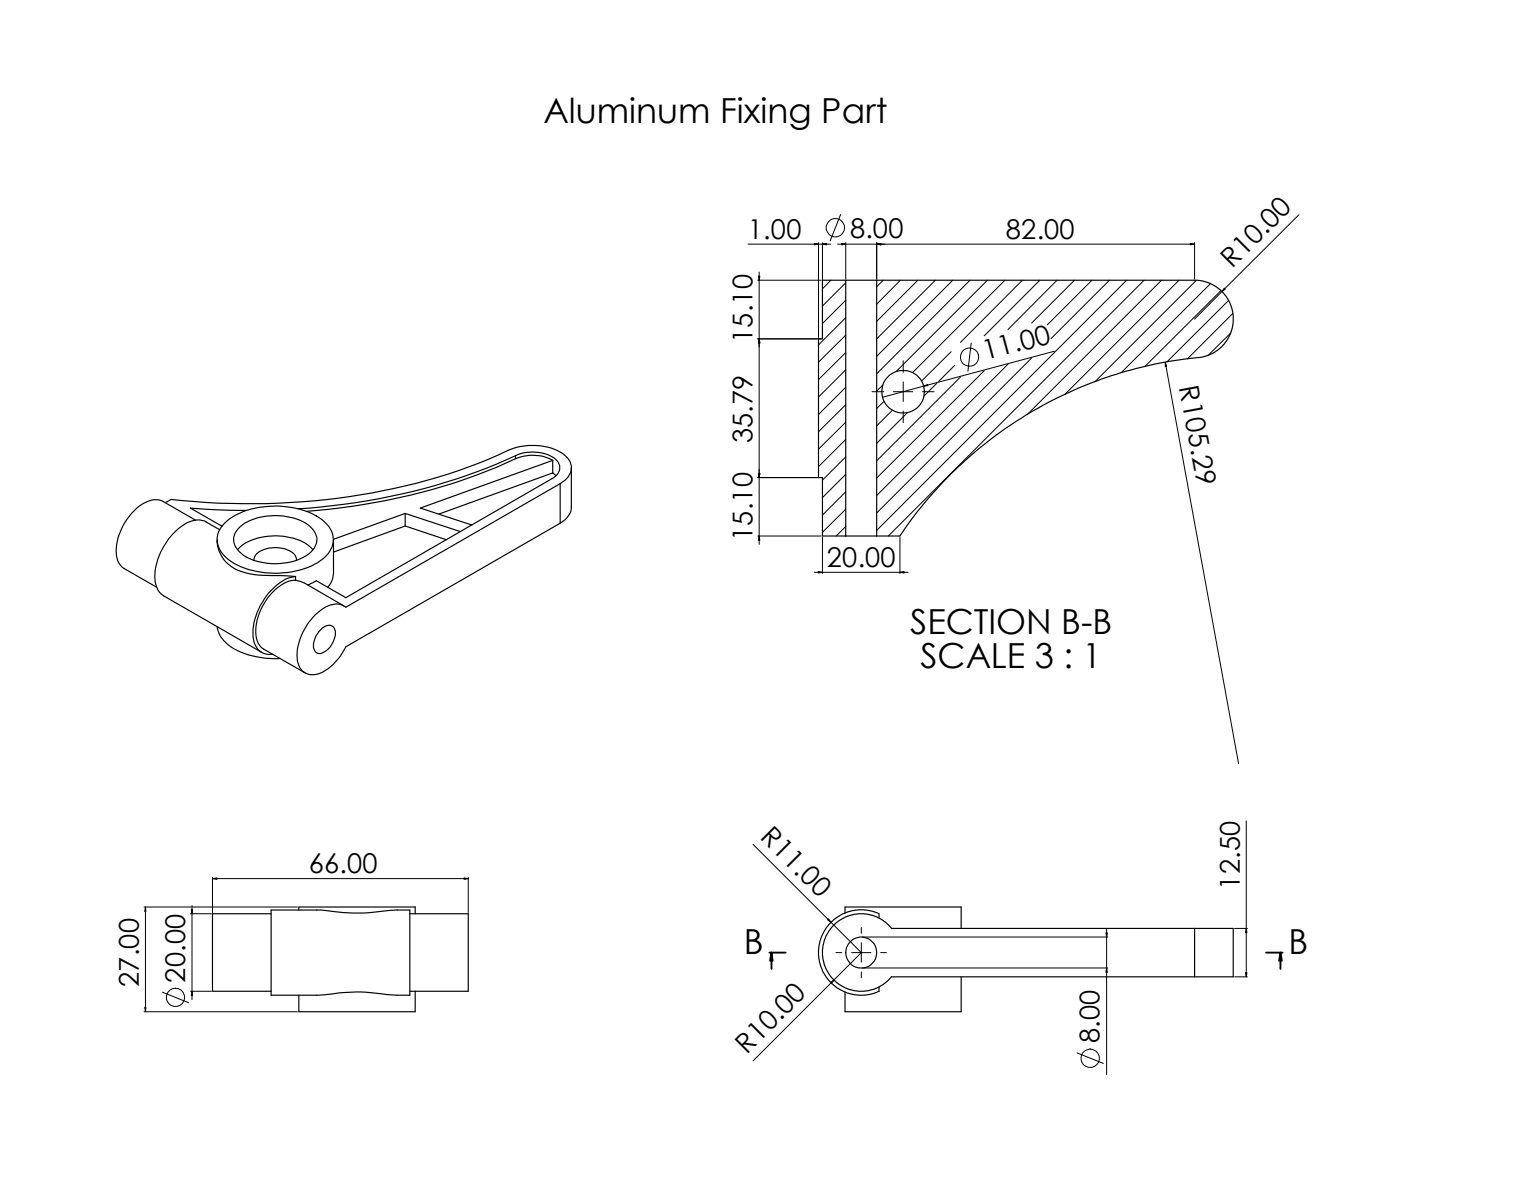
ISO-10303-21;
HEADER;
FILE_DESCRIPTION (('STEP AP214'),
    '1' );
FILE_NAME ('Aluminum Fixing Part.step',
    '2026-10-25T21:42:00',
    ( '' ),
    ( '' ),
    'SwSTEP 2.0',
    'SolidWorks 2025',
    '' );
FILE_SCHEMA (( 'AUTOMOTIVE_DESIGN' ));
ENDSEC;

DATA;
#1=ORIENTED_EDGE ( 'NONE', *, *, #7735, .T. ) ;
#6=CARTESIAN_POINT ( 'NONE',  ( 18.72350467417358288, 2.811787160796888063, 33.16867180916269575 ) ) ;
#84=DIRECTION ( 'NONE',  ( 0.9643627188534427130, 0.000000000000000000, -0.2645837230171117493 ) ) ;
#98=CARTESIAN_POINT ( 'NONE',  ( 4.257384923554910827, 7.250000000000000000, 44.19375250200204164 ) ) ;
#119=( LENGTH_UNIT ( ) NAMED_UNIT ( * ) SI_UNIT ( .MILLI., .METRE. ) );
#157=DIRECTION ( 'NONE',  ( 0.000000000000000000, -1.000000000000000000, 0.000000000000000000 ) ) ;
#171=DIRECTION ( 'NONE',  ( 0.000000000000000000, 0.000000000000000000, 1.000000000000000000 ) ) ;
#189=CARTESIAN_POINT ( 'NONE',  ( 4.257384923554910827, 5.669190722567434726, 44.19375250200204164 ) ) ;
#202=EDGE_LOOP ( 'NONE', ( #15560, #16098, #14916, #31484, #39561 ) ) ;
#206=ORIENTED_EDGE ( 'NONE', *, *, #8749, .F. ) ;
#214=CARTESIAN_POINT ( 'NONE',  ( -2.668805347656625298E-15, -4.500000000000000000, 40.00000000000002132 ) ) ;
#223=VERTEX_POINT ( 'NONE', #2823 ) ;
#248=CARTESIAN_POINT ( 'NONE',  ( 30.00000000000000000, 21.91020392607983780, -13.91584042252958930 ) ) ;
#255=ORIENTED_EDGE ( 'NONE', *, *, #34285, .F. ) ;
#303=ORIENTED_EDGE ( 'NONE', *, *, #35020, .T. ) ;
#331=( NAMED_UNIT ( * ) SI_UNIT ( $, .STERADIAN. ) SOLID_ANGLE_UNIT ( ) );
#338=EDGE_CURVE ( 'NONE', #35065, #41070, #33507, .T. ) ;
#384=LINE ( 'NONE', #32919, #10892 ) ;
#399=CARTESIAN_POINT ( 'NONE',  ( 8.846224670336669149, -14.93588149077679006, 43.47904789183715479 ) ) ;
#437=ORIENTED_EDGE ( 'NONE', *, *, #42084, .T. ) ;
#463=CARTESIAN_POINT ( 'NONE',  ( -26.68952268848979870, -10.75000000000000000, 29.19375250200205230 ) ) ;
#479=ORIENTED_EDGE ( 'NONE', *, *, #8404, .T. ) ;
#515=DIRECTION ( 'NONE',  ( -0.000000000000000000, 1.000000000000000000, -0.000000000000000000 ) ) ;
#522=PRODUCT_CONTEXT ( 'NONE', #9527, 'mechanical' ) ;
#528=EDGE_LOOP ( 'NONE', ( #25720, #24878, #1086, #1385 ) ) ;
#534=EDGE_CURVE ( 'NONE', #29227, #21343, #35976, .T. ) ;
#535=ORIENTED_EDGE ( 'NONE', *, *, #30609, .T. ) ;
#569=VERTEX_POINT ( 'NONE', #13431 ) ;
#579=DIRECTION ( 'NONE',  ( 0.000000000000000000, 1.000000000000000000, 0.000000000000000000 ) ) ;
#623=ORIENTED_EDGE ( 'NONE', *, *, #27491, .F. ) ;
#670=DIRECTION ( 'NONE',  ( 0.000000000000000000, -0.000000000000000000, 1.000000000000000000 ) ) ;
#675=LINE ( 'NONE', #32171, #20640 ) ;
#684=EDGE_CURVE ( 'NONE', #35318, #5713, #28096, .T. ) ;
#732=EDGE_CURVE ( 'NONE', #4073, #42083, #27874, .T. ) ;
#738=VECTOR ( 'NONE', #22456, 1000.000000000000000 ) ;
#761=CARTESIAN_POINT ( 'NONE',  ( 17.89728711128010730, -14.50803179344132410, 35.43499182679077109 ) ) ;
#780=CARTESIAN_POINT ( 'NONE',  ( 13.04894127963215666, -10.75000000000000000, -46.98814490019994139 ) ) ;
#788=ORIENTED_EDGE ( 'NONE', *, *, #20511, .T. ) ;
#802=VERTEX_POINT ( 'NONE', #2351 ) ;
#828=CARTESIAN_POINT ( 'NONE',  ( 15.87547634500077720, -15.42497640701065009, 38.68845844545155188 ) ) ;
#848=DIRECTION ( 'NONE',  ( 1.000000000000000000, 0.000000000000000000, 2.102695122396128930E-16 ) ) ;
#868=CIRCLE ( 'NONE', #30073, 14.99999999999999822 ) ;
#905=EDGE_CURVE ( 'NONE', #16080, #12680, #8463, .T. ) ;
#914=DIRECTION ( 'NONE',  ( 0.000000000000000000, 0.000000000000000000, -1.000000000000000000 ) ) ;
#956=DIRECTION ( 'NONE',  ( 0.000000000000000000, 0.000000000000000000, 1.000000000000000000 ) ) ;
#965=CARTESIAN_POINT ( 'NONE',  ( 18.48006385112488914, -12.48392328919574723, 33.96838569447678680 ) ) ;
#1041=CARTESIAN_POINT ( 'NONE',  ( 4.257384923554910827, 7.250000000000000000, 18.45625250200204448 ) ) ;
#1064=EDGE_LOOP ( 'NONE', ( #30938, #17529, #27633, #33315, #32704 ) ) ;
#1065=CARTESIAN_POINT ( 'NONE',  ( 33.00000000000001421, -4.500000000000000000, 44.00000000000003553 ) ) ;
#1086=ORIENTED_EDGE ( 'NONE', *, *, #29539, .F. ) ;
#1108=CARTESIAN_POINT ( 'NONE',  ( -91.72768752788732627, 1.750000000000001554, -57.39251435732919049 ) ) ;
#1112=ORIENTED_EDGE ( 'NONE', *, *, #1673, .T. ) ;
#1128=CYLINDRICAL_SURFACE ( 'NONE', #31278, 6.999999999999992006 ) ;
#1157=ORIENTED_EDGE ( 'NONE', *, *, #35020, .F. ) ;
#1166=ORIENTED_EDGE ( 'NONE', *, *, #16821, .F. ) ;
#1190=EDGE_CURVE ( 'NONE', #17500, #24287, #25899, .T. ) ;
#1236=CARTESIAN_POINT ( 'NONE',  ( 30.00000000000000000, -9.749999999999998224, -18.08432671081678578 ) ) ;
#1249=LINE ( 'NONE', #36764, #28635 ) ;
#1297=CARTESIAN_POINT ( 'NONE',  ( 4.257384923554909051, 7.250000000000000000, 14.19375250200204341 ) ) ;
#1320=CARTESIAN_POINT ( 'NONE',  ( 14.23381301606215743, -9.749999999999998224, -13.75869656311284217 ) ) ;
#1341=ORIENTED_EDGE ( 'NONE', *, *, #29539, .T. ) ;
#1351=CYLINDRICAL_SURFACE ( 'NONE', #32758, 14.99999999999999822 ) ;
#1361=DIRECTION ( 'NONE',  ( -0.2262442655067632979, 0.000000000000000000, 0.9740705992510528821 ) ) ;
#1385=ORIENTED_EDGE ( 'NONE', *, *, #3747, .F. ) ;
#1399=AXIS2_PLACEMENT_3D ( 'NONE', #38399, #31174, #2036 ) ;
#1431=VERTEX_POINT ( 'NONE', #463 ) ;
#1437=CIRCLE ( 'NONE', #36745, 14.99999999999999822 ) ;
#1474=DIRECTION ( 'NONE',  ( -1.000000000000000000, -0.000000000000000000, -2.102695122396128930E-16 ) ) ;
#1490=DIRECTION ( 'NONE',  ( 0.000000000000000000, -1.000000000000000000, 0.000000000000000000 ) ) ;
#1501=EDGE_CURVE ( 'NONE', #30509, #12679, #675, .T. ) ;
#1549=CIRCLE ( 'NONE', #13787, 6.999999999999992006 ) ;
#1598=DIRECTION ( 'NONE',  ( 0.000000000000000000, -1.000000000000000000, 0.000000000000000000 ) ) ;
#1644=CARTESIAN_POINT ( 'NONE',  ( -10.74261507644508740, 7.250000000000000000, 29.19375250200204874 ) ) ;
#1646=ORIENTED_EDGE ( 'NONE', *, *, #5150, .F. ) ;
#1647=CARTESIAN_POINT ( 'NONE',  ( -33.00000000000002842, -4.500000000000000000, 44.00000000000004263 ) ) ;
#1660=LINE ( 'NONE', #14220, #23405 ) ;
#1667=DIRECTION ( 'NONE',  ( -0.000000000000000000, -1.000000000000000000, -0.000000000000000000 ) ) ;
#1673=EDGE_CURVE ( 'NONE', #41395, #36201, #4074, .T. ) ;
#1675=CARTESIAN_POINT ( 'NONE',  ( -91.72768752788732627, -3.250000000000000444, -57.39251435732919049 ) ) ;
#1678=DIRECTION ( 'NONE',  ( -0.000000000000000000, -1.000000000000000000, -0.000000000000000000 ) ) ;
#1679=CARTESIAN_POINT ( 'NONE',  ( -0.5106722413223524493, -14.95454093630399584, 43.42407850341640341 ) ) ;
#1696=CIRCLE ( 'NONE', #25486, 15.00000000000000000 ) ;
#1709=CARTESIAN_POINT ( 'NONE',  ( 23.34627465269464253, 0.7499999999999997780, -52.99143003003683816 ) ) ;
#1793=EDGE_CURVE ( 'NONE', #15754, #39599, #21910, .T. ) ;
#1796=ORIENTED_EDGE ( 'NONE', *, *, #1673, .F. ) ;
#1814=CARTESIAN_POINT ( 'NONE',  ( 4.257384923554909051, 7.250000000000000000, 29.19375250200204164 ) ) ;
#1821=DIRECTION ( 'NONE',  ( 1.000000000000000000, 0.000000000000000000, 2.102695122396128930E-16 ) ) ;
#1838=ORIENTED_EDGE ( 'NONE', *, *, #21618, .F. ) ;
#1839=ORIENTED_EDGE ( 'NONE', *, *, #14513, .F. ) ;
#1851=EDGE_LOOP ( 'NONE', ( #22250, #25565, #37785, #9057, #37506, #35332 ) ) ;
#1877=FACE_OUTER_BOUND ( 'NONE', #9222, .T. ) ;
#1884=DIRECTION ( 'NONE',  ( 0.000000000000000000, -1.000000000000000000, 0.000000000000000000 ) ) ;
#1931=CARTESIAN_POINT ( 'NONE',  ( -33.00000000000001421, -10.75000000000000000, 30.00000000000003908 ) ) ;
#1939=LINE ( 'NONE', #40862, #7559 ) ;
#1968=PLANE ( 'NONE',  #5767 ) ;
#1980=( GEOMETRIC_REPRESENTATION_CONTEXT ( 3 ) GLOBAL_UNCERTAINTY_ASSIGNED_CONTEXT ( ( #22057 ) ) GLOBAL_UNIT_ASSIGNED_CONTEXT ( ( #119, #13729, #331 ) ) REPRESENTATION_CONTEXT ( 'NONE', 'WORKASPACE' ) );
#1997=ORIENTED_EDGE ( 'NONE', *, *, #3548, .T. ) ;
#1998=AXIS2_PLACEMENT_3D ( 'NONE', #9107, #26127, #9325 ) ;
#2007=ADVANCED_FACE ( 'NONE', ( #9800 ), #22758, .F. ) ;
#2036=DIRECTION ( 'NONE',  ( 0.000000000000000000, 0.000000000000000000, -1.000000000000000000 ) ) ;
#2073=ADVANCED_FACE ( 'NONE', ( #7870, #20838 ), #16801, .T. ) ;
#2124=VECTOR ( 'NONE', #16063, 1000.000000000000000 ) ;
#2173=VECTOR ( 'NONE', #32065, 1000.000000000000000 ) ;
#2222=DIRECTION ( 'NONE',  ( 0.000000000000000000, 1.000000000000000000, 0.000000000000000000 ) ) ;
#2268=VECTOR ( 'NONE', #13230, 1000.000000000000000 ) ;
#2273=AXIS2_PLACEMENT_3D ( 'NONE', #35262, #37618, #15075 ) ;
#2285=CARTESIAN_POINT ( 'NONE',  ( 19.25738492355490550, 7.250000000000000000, 29.19375250200203453 ) ) ;
#2310=VERTEX_POINT ( 'NONE', #23315 ) ;
#2351=CARTESIAN_POINT ( 'NONE',  ( 4.257384923554909051, 7.250000000000000000, 14.19375250200204341 ) ) ;
#2361=ORIENTED_EDGE ( 'NONE', *, *, #9207, .T. ) ;
#2370=EDGE_CURVE ( 'NONE', #42083, #8731, #12533, .T. ) ;
#2371=ORIENTED_EDGE ( 'NONE', *, *, #22389, .F. ) ;
#2384=CIRCLE ( 'NONE', #17332, 6.999999999999992006 ) ;
#2398=VERTEX_POINT ( 'NONE', #7417 ) ;
#2411=CARTESIAN_POINT ( 'NONE',  ( -1.027389493830893750E-15, -10.75000000000000000, 32.19375250200204874 ) ) ;
#2459=CARTESIAN_POINT ( 'NONE',  ( 4.257384923554909051, -5.749999999999999112, 29.19375250200204164 ) ) ;
#2480=CARTESIAN_POINT ( 'NONE',  ( -33.00000000000002842, -4.500000000000000000, 49.99999999999999289 ) ) ;
#2501=CARTESIAN_POINT ( 'NONE',  ( 30.00000000000001776, -5.749999999999999112, 29.19375250200203098 ) ) ;
#2556=DIRECTION ( 'NONE',  ( -2.102695122396129176E-16, 0.000000000000000000, 1.000000000000000000 ) ) ;
#2559=ORIENTED_EDGE ( 'NONE', *, *, #34285, .T. ) ;
#2569=ORIENTED_EDGE ( 'NONE', *, *, #25405, .T. ) ;
#2571=ORIENTED_EDGE ( 'NONE', *, *, #13609, .T. ) ;
#2611=AXIS2_PLACEMENT_3D ( 'NONE', #19606, #17060, #3244 ) ;
#2612=ORIENTED_EDGE ( 'NONE', *, *, #25476, .F. ) ;
#2636=FACE_OUTER_BOUND ( 'NONE', #15761, .T. ) ;
#2667=DIRECTION ( 'NONE',  ( -2.102695122396128190E-16, 0.000000000000000000, 1.000000000000000000 ) ) ;
#2678=ORIENTED_EDGE ( 'NONE', *, *, #12925, .T. ) ;
#2708=CYLINDRICAL_SURFACE ( 'NONE', #30544, 9.999999999999994671 ) ;
#2721=CARTESIAN_POINT ( 'NONE',  ( -10.23396330418008304, -13.04708509534837191, 33.07144372220358974 ) ) ;
#2728=EDGE_CURVE ( 'NONE', #29182, #24045, #1660, .T. ) ;
#2734=ORIENTED_EDGE ( 'NONE', *, *, #24119, .F. ) ;
#2784=CARTESIAN_POINT ( 'NONE',  ( -12.28065031820329089, -3.250000000000000444, 16.19629439043522723 ) ) ;
#2801=AXIS2_PLACEMENT_3D ( 'NONE', #10030, #19387, #38743 ) ;
#2823=CARTESIAN_POINT ( 'NONE',  ( -17.89728711128011795, -10.75000000000000000, 30.94806650488419564 ) ) ;
#2837=EDGE_CURVE ( 'NONE', #12680, #28256, #28822, .T. ) ;
#2841=FACE_OUTER_BOUND ( 'NONE', #39716, .T. ) ;
#2864=LINE ( 'NONE', #15854, #11765 ) ;
#2881=CARTESIAN_POINT ( 'NONE',  ( 23.34627465269464253, 0.7499999999999997780, -52.99143003003683816 ) ) ;
#2916=CARTESIAN_POINT ( 'NONE',  ( 17.89728711128010730, -4.500000000000000000, 40.00000000000002842 ) ) ;
#2921=DIRECTION ( 'NONE',  ( -0.000000000000000000, -1.000000000000000000, -0.000000000000000000 ) ) ;
#2922=DIRECTION ( 'NONE',  ( -1.000000000000000000, 0.000000000000000000, -2.102695122396128930E-16 ) ) ;
#2952=CARTESIAN_POINT ( 'NONE',  ( -11.21606888246744127, 0.7499999999999997780, 29.19375250200204519 ) ) ;
#2967=CARTESIAN_POINT ( 'NONE',  ( 2.309751567486731272, 5.717580681526216679, 44.07476052617663242 ) ) ;
#3004=VERTEX_POINT ( 'NONE', #28229 ) ;
#3037=CIRCLE ( 'NONE', #13903, 4.000000000000003553 ) ;
#3043=ADVANCED_FACE ( 'NONE', ( #19081 ), #31211, .T. ) ;
#3084=DIRECTION ( 'NONE',  ( -3.154042683594197586E-16, 0.000000000000000000, 1.000000000000000000 ) ) ;
#3090=CIRCLE ( 'NONE', #25506, 15.00000000000000000 ) ;
#3100=EDGE_LOOP ( 'NONE', ( #31440, #6346 ) ) ;
#3143=ORIENTED_EDGE ( 'NONE', *, *, #6114, .T. ) ;
#3153=CARTESIAN_POINT ( 'NONE',  ( 4.257384923554909051, 7.250000000000000000, 14.19375250200204341 ) ) ;
#3166=CARTESIAN_POINT ( 'NONE',  ( 17.75723580862730699, 5.647643056288242924, 35.74106662540655321 ) ) ;
#3169=VECTOR ( 'NONE', #5542, 1000.000000000000000 ) ;
#3204=CARTESIAN_POINT ( 'NONE',  ( 18.90801972032829426, 2.033323918614180492, 32.42059318208459473 ) ) ;
#3221=EDGE_CURVE ( 'NONE', #1431, #39128, #27504, .T. ) ;
#3244=DIRECTION ( 'NONE',  ( 0.000000000000000000, 0.000000000000000000, 1.000000000000000000 ) ) ;
#3287=DIRECTION ( 'NONE',  ( 2.768405754343413644E-16, 0.000000000000000000, 1.000000000000000000 ) ) ;
#3294=DIRECTION ( 'NONE',  ( 0.000000000000000000, 0.000000000000000000, -1.000000000000000000 ) ) ;
#3341=VECTOR ( 'NONE', #1678, 1000.000000000000000 ) ;
#3355=LINE ( 'NONE', #3153, #25287 ) ;
#3359=VECTOR ( 'NONE', #24512, 1000.000000000000000 ) ;
#3434=DIRECTION ( 'NONE',  ( 0.000000000000000000, 1.000000000000000000, 0.000000000000000000 ) ) ;
#3460=CYLINDRICAL_SURFACE ( 'NONE', #41823, 6.999999999999992006 ) ;
#3508=ORIENTED_EDGE ( 'NONE', *, *, #26473, .F. ) ;
#3509=ORIENTED_EDGE ( 'NONE', *, *, #34672, .T. ) ;
#3534=CIRCLE ( 'NONE', #33420, 6.999999999999992006 ) ;
#3539=CIRCLE ( 'NONE', #30021, 9.999999999999973355 ) ;
#3548=EDGE_CURVE ( 'NONE', #13653, #11217, #2384, .T. ) ;
#3555=CARTESIAN_POINT ( 'NONE',  ( 29.99999999999999645, 1.749999999999999778, -45.99999999999998579 ) ) ;
#3583=CARTESIAN_POINT ( 'NONE',  ( 9.856488012272384580, -15.05078906327959309, 43.11419007114952962 ) ) ;
#3595=CARTESIAN_POINT ( 'NONE',  ( 4.257384923554909051, -19.75000000000000000, 29.19375250200204164 ) ) ;
#3620=AXIS2_PLACEMENT_3D ( 'NONE', #3743, #29691, #17149 ) ;
#3624=VECTOR ( 'NONE', #5285, 1000.000000000000000 ) ;
#3713=EDGE_LOOP ( 'NONE', ( #24939, #26334, #1796, #17799, #33123 ) ) ;
#3717=ORIENTED_EDGE ( 'NONE', *, *, #22740, .F. ) ;
#3725=AXIS2_PLACEMENT_3D ( 'NONE', #1814, #14794, #28175 ) ;
#3740=AXIS2_PLACEMENT_3D ( 'NONE', #13581, #26565, #22945 ) ;
#3743=CARTESIAN_POINT ( 'NONE',  ( 29.99999999999999645, -5.749999999999999112, -45.99999999999998579 ) ) ;
#3747=EDGE_CURVE ( 'NONE', #4073, #35992, #27248, .T. ) ;
#3822=CARTESIAN_POINT ( 'NONE',  ( 30.00000000000001776, 1.749999999999999778, 29.19375250200203098 ) ) ;
#3823=VECTOR ( 'NONE', #4627, 1000.000000000000000 ) ;
#3828=B_SPLINE_CURVE_WITH_KNOTS ( 'NONE', 3,
 ( #41475, #19546, #39107, #38489, #12539, #25307, #22524, #25525, #35917, #29110, #32723, #38696, #9135, #22949, #5944, #41684, #32315, #15958, #35719, #32518, #6367, #9351, #26156, #19341, #25943, #9785, #2967, #28907, #35294, #189 ),
 .UNSPECIFIED., .F., .F.,
 ( 4, 2, 2, 2, 2, 2, 2, 2, 2, 2, 2, 2, 2, 2, 4 ),
 ( 0.000000000000000000, 0.002908868141953183800, 0.003636085177441482786, 0.004363302212929782639, 0.005817736283906382345, 0.007272170354882981184, 0.008726604425859580891, 0.01018103849683617973, 0.01163547256781278204, 0.01308990663878938088, 0.01454434070976597972, 0.01745320885171916872, 0.02036207699367235946, 0.02181651106464895309, 0.02327094513562554326 ),
 .UNSPECIFIED. ) ;
#3833=EDGE_CURVE ( 'NONE', #802, #24819, #20860, .T. ) ;
#3848=DIRECTION ( 'NONE',  ( 0.000000000000000000, 0.000000000000000000, -1.000000000000000000 ) ) ;
#3860=CARTESIAN_POINT ( 'NONE',  ( 19.25738492355490550, -5.749999999999999112, 29.19375250200203453 ) ) ;
#3874=LINE ( 'NONE', #36190, #39548 ) ;
#3914=EDGE_LOOP ( 'NONE', ( #16197, #33119, #31693, #28161, #7191, #5153 ) ) ;
#3969=EDGE_LOOP ( 'NONE', ( #20843, #22757, #4098, #255 ) ) ;
#3995=PLANE ( 'NONE',  #40031 ) ;
#4000=CIRCLE ( 'NONE', #30481, 105.2919410404669520 ) ;
#4009=ADVANCED_FACE ( 'NONE', ( #34655 ), #12103, .F. ) ;
#4073=VERTEX_POINT ( 'NONE', #38485 ) ;
#4074=LINE ( 'NONE', #17058, #18601 ) ;
#4093=CARTESIAN_POINT ( 'NONE',  ( 22.99999999999999645, -5.749999999999999112, -45.99999999999998579 ) ) ;
#4098=ORIENTED_EDGE ( 'NONE', *, *, #21660, .T. ) ;
#4123=VERTEX_POINT ( 'NONE', #25095 ) ;
#4128=DIRECTION ( 'NONE',  ( 0.000000000000000000, 0.000000000000000000, 1.000000000000000000 ) ) ;
#4146=CARTESIAN_POINT ( 'NONE',  ( -33.00000000000001421, 1.750000000000001554, 30.00000000000003908 ) ) ;
#4163=DIRECTION ( 'NONE',  ( -0.000000000000000000, -1.000000000000000000, -0.000000000000000000 ) ) ;
#4178=AXIS2_PLACEMENT_3D ( 'NONE', #9768, #19117, #22301 ) ;
#4187=CARTESIAN_POINT ( 'NONE',  ( 32.99999999999999289, -10.75000000000000000, -45.99999999999999289 ) ) ;
#4234=AXIS2_PLACEMENT_3D ( 'NONE', #7078, #24104, #7294 ) ;
#4270=CARTESIAN_POINT ( 'NONE',  ( -1.027389493830893947E-15, 1.750000000000001554, 32.19375250200204874 ) ) ;
#4293=ORIENTED_EDGE ( 'NONE', *, *, #19638, .T. ) ;
#4294=EDGE_CURVE ( 'NONE', #36380, #32144, #39768, .T. ) ;
#4305=VECTOR ( 'NONE', #39253, 1000.000000000000000 ) ;
#4311=EDGE_CURVE ( 'NONE', #18130, #33817, #23660, .T. ) ;
#4313=LINE ( 'NONE', #36206, #40902 ) ;
#4352=ORIENTED_EDGE ( 'NONE', *, *, #12147, .F. ) ;
#4354=ORIENTED_EDGE ( 'NONE', *, *, #684, .T. ) ;
#4361=CARTESIAN_POINT ( 'NONE',  ( 18.73745248760390680, -11.81953870135891727, 33.15033124357624672 ) ) ;
#4381=CARTESIAN_POINT ( 'NONE',  ( -91.72768752788732627, -5.749999999999999112, -57.39251435732919049 ) ) ;
#4419=EDGE_LOOP ( 'NONE', ( #535, #13244, #33812, #10641, #19619, #18898 ) ) ;
#4424=ORIENTED_EDGE ( 'NONE', *, *, #14671, .F. ) ;
#4431=DIRECTION ( 'NONE',  ( -0.000000000000000000, -1.000000000000000000, -0.000000000000000000 ) ) ;
#4454=DIRECTION ( 'NONE',  ( 0.000000000000000000, 1.000000000000000000, 0.000000000000000000 ) ) ;
#4471=AXIS2_PLACEMENT_3D ( 'NONE', #15487, #22071, #41430 ) ;
#4487=CARTESIAN_POINT ( 'NONE',  ( 23.34627465269464253, -5.749999999999999112, -52.99143003003683816 ) ) ;
#4524=DIRECTION ( 'NONE',  ( 0.000000000000000000, 0.000000000000000000, 1.000000000000000000 ) ) ;
#4553=EDGE_CURVE ( 'NONE', #5666, #24045, #3090, .T. ) ;
#4597=DIRECTION ( 'NONE',  ( -0.000000000000000000, 1.000000000000000000, -0.000000000000000000 ) ) ;
#4627=DIRECTION ( 'NONE',  ( 2.102695122396128930E-16, 0.000000000000000000, -1.000000000000000000 ) ) ;
#4645=LINE ( 'NONE', #7208, #21837 ) ;
#4656=DIRECTION ( 'NONE',  ( -1.000000000000000000, -0.000000000000000000, -2.102695122396128930E-16 ) ) ;
#4659=DIRECTION ( 'NONE',  ( -0.9643627188534427130, 0.000000000000000000, 0.2645837230171119159 ) ) ;
#4661=CARTESIAN_POINT ( 'NONE',  ( -4.794472690475274135, -15.44843424009357769, 41.19453516596701803 ) ) ;
#4664=DIRECTION ( 'NONE',  ( 0.000000000000000000, 0.000000000000000000, -1.000000000000000000 ) ) ;
#4678=CIRCLE ( 'NONE', #23723, 14.99999999999999822 ) ;
#4692=DIRECTION ( 'NONE',  ( -0.000000000000000000, 1.000000000000000000, -0.000000000000000000 ) ) ;
#4720=ORIENTED_EDGE ( 'NONE', *, *, #32766, .T. ) ;
#4772=EDGE_LOOP ( 'NONE', ( #4354, #20575, #41192, #2678 ) ) ;
#4776=PRODUCT_DEFINITION_SHAPE ( 'NONE', 'NONE',  #40299 ) ;
#4811=AXIS2_PLACEMENT_3D ( 'NONE', #4985, #17759, #17550 ) ;
#4821=EDGE_CURVE ( 'NONE', #24046, #39599, #868, .T. ) ;
#4830=VECTOR ( 'NONE', #24916, 1000.000000000000000 ) ;
#4836=FACE_BOUND ( 'NONE', #10514, .T. ) ;
#4926=LINE ( 'NONE', #11311, #23117 ) ;
#4954=LINE ( 'NONE', #33691, #35491 ) ;
#4957=EDGE_CURVE ( 'NONE', #18534, #41673, #17148, .T. ) ;
#4985=CARTESIAN_POINT ( 'NONE',  ( 11.02911845508759470, 21.91020392607983780, -8.710966395423659137 ) ) ;
#5002=AXIS2_PLACEMENT_3D ( 'NONE', #3595, #20196, #16588 ) ;
#5014=ORIENTED_EDGE ( 'NONE', *, *, #19271, .F. ) ;
#5038=CIRCLE ( 'NONE', #26085, 108.2919410404669378 ) ;
#5039=EDGE_LOOP ( 'NONE', ( #14097, #17029, #28884, #38406, #6291, #41242, #18423, #5446, #35939, #303, #35636 ) ) ;
#5073=CARTESIAN_POINT ( 'NONE',  ( -6.589185986107628956, -15.49669818324776216, 39.56620216159959114 ) ) ;
#5121=PLANE ( 'NONE',  #8191 ) ;
#5134=ORIENTED_EDGE ( 'NONE', *, *, #37233, .F. ) ;
#5143=VECTOR ( 'NONE', #16022, 1000.000000000000000 ) ;
#5150=EDGE_CURVE ( 'NONE', #28829, #28670, #38881, .T. ) ;
#5153=ORIENTED_EDGE ( 'NONE', *, *, #2837, .T. ) ;
#5241=ORIENTED_EDGE ( 'NONE', *, *, #14353, .T. ) ;
#5270=DIRECTION ( 'NONE',  ( -2.102695122396129176E-16, 0.000000000000000000, 1.000000000000000000 ) ) ;
#5282=CARTESIAN_POINT ( 'NONE',  ( 3.285248659299954799, -14.66919072256743917, 44.19375250200204164 ) ) ;
#5285=DIRECTION ( 'NONE',  ( -0.000000000000000000, 1.000000000000000000, -0.000000000000000000 ) ) ;
#5336=ORIENTED_EDGE ( 'NONE', *, *, #39509, .T. ) ;
#5338=VERTEX_POINT ( 'NONE', #36740 ) ;
#5339=VECTOR ( 'NONE', #38136, 1000.000000000000000 ) ;
#5382=VECTOR ( 'NONE', #12046, 1000.000000000000000 ) ;
#5419=CARTESIAN_POINT ( 'NONE',  ( -33.00000000000001421, -10.75000000000000000, 32.19375250200204164 ) ) ;
#5430=CIRCLE ( 'NONE', #12906, 14.99999999999999822 ) ;
#5442=CARTESIAN_POINT ( 'NONE',  ( 14.23381301606215921, -3.250000000000000444, -13.75869656311284217 ) ) ;
#5444=AXIS2_PLACEMENT_3D ( 'NONE', #18016, #11014, #40768 ) ;
#5446=ORIENTED_EDGE ( 'NONE', *, *, #36682, .T. ) ;
#5481=DIRECTION ( 'NONE',  ( -2.102695122396128930E-16, 0.000000000000000000, 1.000000000000000000 ) ) ;
#5498=LINE ( 'NONE', #37620, #14214 ) ;
#5542=DIRECTION ( 'NONE',  ( -0.000000000000000000, -1.000000000000000000, -0.000000000000000000 ) ) ;
#5548=LINE ( 'NONE', #31490, #41509 ) ;
#5583=DIRECTION ( 'NONE',  ( -0.000000000000000000, 1.000000000000000000, -0.000000000000000000 ) ) ;
#5589=ORIENTED_EDGE ( 'NONE', *, *, #38937, .F. ) ;
#5594=CARTESIAN_POINT ( 'NONE',  ( 29.99999999999999645, -5.749999999999999112, -45.99999999999998579 ) ) ;
#5605=B_SPLINE_CURVE_WITH_KNOTS ( 'NONE', 3,
 ( #10739, #10955, #4361, #965, #26913, #33718, #36477, #24154 ),
 .UNSPECIFIED., .F., .F.,
 ( 4, 2, 2, 4 ),
 ( 1.734723475976806902E-18, 0.002164095738853550385, 0.003246143608280325360, 0.004328191477707100769 ),
 .UNSPECIFIED. ) ;
#5606=ADVANCED_FACE ( 'NONE', ( #17310 ), #1351, .T. ) ;
#5609=AXIS2_PLACEMENT_3D ( 'NONE', #6209, #28953, #16623 ) ;
#5611=ORIENTED_EDGE ( 'NONE', *, *, #16154, .T. ) ;
#5666=VERTEX_POINT ( 'NONE', #39625 ) ;
#5682=ADVANCED_FACE ( 'NONE', ( #30909 ), #28123, .F. ) ;
#5694=DIRECTION ( 'NONE',  ( 0.2645837230171118049, -0.000000000000000000, 0.9643627188534428241 ) ) ;
#5696=CARTESIAN_POINT ( 'NONE',  ( 30.00000000000000000, 21.91020392607983780, -13.91584042252958930 ) ) ;
#5701=ORIENTED_EDGE ( 'NONE', *, *, #24096, .T. ) ;
#5704=VECTOR ( 'NONE', #4656, 1000.000000000000000 ) ;
#5710=CARTESIAN_POINT ( 'NONE',  ( 23.34627465269464253, -9.749999999999998224, -52.99143003003683816 ) ) ;
#5713=VERTEX_POINT ( 'NONE', #14948 ) ;
#5719=DIRECTION ( 'NONE',  ( -0.2262442655067632979, 0.000000000000000000, 0.9740705992510528821 ) ) ;
#5728=ORIENTED_EDGE ( 'NONE', *, *, #18907, .T. ) ;
#5731=CIRCLE ( 'NONE', #9125, 6.999999999999992006 ) ;
#5767=AXIS2_PLACEMENT_3D ( 'NONE', #34095, #14753, #30912 ) ;
#5774=CARTESIAN_POINT ( 'NONE',  ( 30.00000000000000355, 0.7499999999999997780, -18.08432671081678578 ) ) ;
#5824=EDGE_LOOP ( 'NONE', ( #39238, #30888, #31189, #5701 ) ) ;
#5827=CARTESIAN_POINT ( 'NONE',  ( 4.257384923554909051, 7.250000000000000000, 39.93125250200203880 ) ) ;
#5852=CARTESIAN_POINT ( 'NONE',  ( -7.654597068132068207E-16, -10.75000000000000000, 30.94806650488419919 ) ) ;
#5858=ORIENTED_EDGE ( 'NONE', *, *, #34672, .F. ) ;
#5916=CARTESIAN_POINT ( 'NONE',  ( 19.25738492355490550, -3.250000000000000444, 29.19375250200203453 ) ) ;
#5928=EDGE_CURVE ( 'NONE', #11308, #15664, #30747, .T. ) ;
#5931=CARTESIAN_POINT ( 'NONE',  ( 13.57193988865721224, 6.467008697123466376, 40.97308721238449181 ) ) ;
#5944=CARTESIAN_POINT ( 'NONE',  ( -7.553706683214575612, 6.397171164914930763, 38.45311005288014172 ) ) ;
#5962=ORIENTED_EDGE ( 'NONE', *, *, #29578, .F. ) ;
#6000=CARTESIAN_POINT ( 'NONE',  ( 4.257384923554909051, 7.250000000000000000, 34.69375250200203453 ) ) ;
#6017=DIRECTION ( 'NONE',  ( -0.000000000000000000, 1.000000000000000000, -0.000000000000000000 ) ) ;
#6030=FACE_OUTER_BOUND ( 'NONE', #25581, .T. ) ;
#6078=ORIENTED_EDGE ( 'NONE', *, *, #19638, .F. ) ;
#6098=DIRECTION ( 'NONE',  ( 0.9966624141706600382, 0.000000000000000000, -0.08163352362547933450 ) ) ;
#6099=CARTESIAN_POINT ( 'NONE',  ( -26.68952268848979870, -5.749999999999999112, 29.19375250200205230 ) ) ;
#6114=EDGE_CURVE ( 'NONE', #13500, #28670, #39151, .T. ) ;
#6118=DIRECTION ( 'NONE',  ( 0.000000000000000000, 0.000000000000000000, -1.000000000000000000 ) ) ;
#6134=AXIS2_PLACEMENT_3D ( 'NONE', #42013, #13694, #37100 ) ;
#6140=CARTESIAN_POINT ( 'NONE',  ( 16.52986725026255854, 6.304568274278368634, 37.84703255120420806 ) ) ;
#6199=CIRCLE ( 'NONE', #25945, 10.00000000000000178 ) ;
#6209=CARTESIAN_POINT ( 'NONE',  ( -33.00000000000002132, -4.500000000000000000, 40.00000000000001421 ) ) ;
#6291=ORIENTED_EDGE ( 'NONE', *, *, #30284, .T. ) ;
#6310=PRODUCT_DEFINITION_CONTEXT ( 'detailed design', #32061, 'design' ) ;
#6314=DIRECTION ( 'NONE',  ( -1.000000000000000000, -0.000000000000000000, 3.672050975999536567E-16 ) ) ;
#6315=DIRECTION ( 'NONE',  ( -3.154042683594197586E-16, 0.000000000000000000, 1.000000000000000000 ) ) ;
#6339=FACE_OUTER_BOUND ( 'NONE', #39927, .T. ) ;
#6341=DIRECTION ( 'NONE',  ( -0.000000000000000000, 1.000000000000000000, -0.000000000000000000 ) ) ;
#6342=AXIS2_PLACEMENT_3D ( 'NONE', #28177, #14378, #34560 ) ;
#6346=ORIENTED_EDGE ( 'NONE', *, *, #32104, .F. ) ;
#6367=CARTESIAN_POINT ( 'NONE',  ( -4.384195450815247419, 6.405474307964317937, 41.46394284326546398 ) ) ;
#6388=ORIENTED_EDGE ( 'NONE', *, *, #29181, .T. ) ;
#6397=ORIENTED_EDGE ( 'NONE', *, *, #13197, .T. ) ;
#6453=CYLINDRICAL_SURFACE ( 'NONE', #20095, 5.499999999999991118 ) ;
#6493=DIRECTION ( 'NONE',  ( -0.2262442655067632979, 0.000000000000000000, 0.9740705992510528821 ) ) ;
#6512=CARTESIAN_POINT ( 'NONE',  ( -3.509883396615080222E-15, -4.500000000000000000, 44.00000000000004263 ) ) ;
#6560=EDGE_CURVE ( 'NONE', #13232, #2398, #3828, .T. ) ;
#6565=VECTOR ( 'NONE', #5719, 1000.000000000000114 ) ;
#6587=FACE_OUTER_BOUND ( 'NONE', #19362, .T. ) ;
#6598=LINE ( 'NONE', #19564, #20522 ) ;
#6612=ORIENTED_EDGE ( 'NONE', *, *, #9872, .F. ) ;
#6643=ORIENTED_EDGE ( 'NONE', *, *, #29531, .T. ) ;
#6726=CARTESIAN_POINT ( 'NONE',  ( -11.21606888246744127, -9.749999999999998224, 29.19375250200204519 ) ) ;
#6746=DIRECTION ( 'NONE',  ( -0.000000000000000000, 1.000000000000000000, -0.000000000000000000 ) ) ;
#6754=VECTOR ( 'NONE', #20752, 1000.000000000000000 ) ;
#6766=CARTESIAN_POINT ( 'NONE',  ( -26.68952268848979870, -3.250000000000000444, 29.19375250200205230 ) ) ;
#6797=ORIENTED_EDGE ( 'NONE', *, *, #22562, .F. ) ;
#6846=FACE_OUTER_BOUND ( 'NONE', #36750, .T. ) ;
#6882=FACE_OUTER_BOUND ( 'NONE', #27169, .T. ) ;
#6887=CARTESIAN_POINT ( 'NONE',  ( 29.99999999999999645, -5.749999999999999112, -45.99999999999998579 ) ) ;
#6969=ADVANCED_FACE ( 'NONE', ( #20543 ), #36706, .T. ) ;
#6981=AXIS2_PLACEMENT_3D ( 'NONE', #37524, #40922, #24981 ) ;
#7013=LINE ( 'NONE', #17446, #21701 ) ;
#7060=CARTESIAN_POINT ( 'NONE',  ( 13.04894127963215666, 1.750000000000001554, -46.98814490019994139 ) ) ;
#7062=DIRECTION ( 'NONE',  ( -1.000000000000000000, 0.000000000000000000, 3.672050975999536567E-16 ) ) ;
#7078=CARTESIAN_POINT ( 'NONE',  ( 4.257384923554909051, 0.8500000000000017542, 29.19375250200204164 ) ) ;
#7110=ORIENTED_EDGE ( 'NONE', *, *, #1190, .T. ) ;
#7120=DIRECTION ( 'NONE',  ( -0.000000000000000000, -1.000000000000000000, -0.000000000000000000 ) ) ;
#7122=ORIENTED_EDGE ( 'NONE', *, *, #35786, .T. ) ;
#7141=EDGE_CURVE ( 'NONE', #28256, #13232, #36884, .T. ) ;
#7176=FACE_OUTER_BOUND ( 'NONE', #33382, .T. ) ;
#7191=ORIENTED_EDGE ( 'NONE', *, *, #27491, .T. ) ;
#7208=CARTESIAN_POINT ( 'NONE',  ( 30.00000000000000000, 0.7500000000000006661, -13.91584042252958930 ) ) ;
#7232=EDGE_CURVE ( 'NONE', #39544, #34649, #21753, .T. ) ;
#7268=EDGE_CURVE ( 'NONE', #33170, #41490, #25378, .T. ) ;
#7294=DIRECTION ( 'NONE',  ( 0.000000000000000000, 0.000000000000000000, 1.000000000000000000 ) ) ;
#7315=ADVANCED_FACE ( 'NONE', ( #22378, #34517 ), #35357, .F. ) ;
#7337=VERTEX_POINT ( 'NONE', #25166 ) ;
#7338=ORIENTED_EDGE ( 'NONE', *, *, #6560, .F. ) ;
#7361=LINE ( 'NONE', #23540, #13143 ) ;
#7396=VERTEX_POINT ( 'NONE', #9200 ) ;
#7417=CARTESIAN_POINT ( 'NONE',  ( 4.257384923554910827, 5.669190722567434726, 44.19375250200204164 ) ) ;
#7419=CARTESIAN_POINT ( 'NONE',  ( 5.704749963857062234, -14.69140052472006985, 44.14097145204375749 ) ) ;
#7446=ORIENTED_EDGE ( 'NONE', *, *, #42084, .F. ) ;
#7491=ORIENTED_EDGE ( 'NONE', *, *, #1793, .F. ) ;
#7535=VERTEX_POINT ( 'NONE', #9580 ) ;
#7558=DIRECTION ( 'NONE',  ( 0.000000000000000000, 1.000000000000000000, 0.000000000000000000 ) ) ;
#7559=VECTOR ( 'NONE', #41080, 1000.000000000000000 ) ;
#7570=DIRECTION ( 'NONE',  ( 0.000000000000000000, 0.000000000000000000, -1.000000000000000000 ) ) ;
#7618=CARTESIAN_POINT ( 'NONE',  ( 30.00000000000000000, 21.91020392607983780, -18.08432671081678578 ) ) ;
#7622=AXIS2_PLACEMENT_3D ( 'NONE', #23223, #6017, #18994 ) ;
#7652=DIRECTION ( 'NONE',  ( -0.000000000000000000, 1.000000000000000000, -0.000000000000000000 ) ) ;
#7659=AXIS2_PLACEMENT_3D ( 'NONE', #22668, #39233, #32241 ) ;
#7660=ORIENTED_EDGE ( 'NONE', *, *, #8749, .T. ) ;
#7700=ORIENTED_EDGE ( 'NONE', *, *, #4553, .F. ) ;
#7735=EDGE_CURVE ( 'NONE', #28095, #11217, #37869, .T. ) ;
#7749=EDGE_LOOP ( 'NONE', ( #12781, #11408 ) ) ;
#7817=CIRCLE ( 'NONE', #31563, 4.000000000000003553 ) ;
#7827=ORIENTED_EDGE ( 'NONE', *, *, #30501, .T. ) ;
#7861=DIRECTION ( 'NONE',  ( 0.000000000000000000, 0.000000000000000000, -1.000000000000000000 ) ) ;
#7870=FACE_OUTER_BOUND ( 'NONE', #202, .T. ) ;
#7908=FACE_OUTER_BOUND ( 'NONE', #37627, .T. ) ;
#7912=ORIENTED_EDGE ( 'NONE', *, *, #31833, .F. ) ;
#7915=CARTESIAN_POINT ( 'NONE',  ( 22.99999999999999645, 1.750000000000001554, -45.99999999999998579 ) ) ;
#7927=ORIENTED_EDGE ( 'NONE', *, *, #8080, .T. ) ;
#7935=ORIENTED_EDGE ( 'NONE', *, *, #8370, .F. ) ;
#8002=FACE_OUTER_BOUND ( 'NONE', #30574, .T. ) ;
#8026=DIRECTION ( 'NONE',  ( 0.2262442655067633257, 0.000000000000000000, -0.9740705992510528821 ) ) ;
#8027=EDGE_CURVE ( 'NONE', #39128, #13653, #3534, .T. ) ;
#8037=EDGE_CURVE ( 'NONE', #33817, #37325, #40396, .T. ) ;
#8052=AXIS2_PLACEMENT_3D ( 'NONE', #7915, #20464, #27059 ) ;
#8061=CARTESIAN_POINT ( 'NONE',  ( -5.548789800779364789, -15.50540173716706605, 40.58595101821124729 ) ) ;
#8080=EDGE_CURVE ( 'NONE', #39224, #19770, #28248, .T. ) ;
#8119=VECTOR ( 'NONE', #32035, 1000.000000000000000 ) ;
#8191=AXIS2_PLACEMENT_3D ( 'NONE', #22489, #24698, #11295 ) ;
#8231=EDGE_CURVE ( 'NONE', #18130, #16080, #28066, .T. ) ;
#8261=ORIENTED_EDGE ( 'NONE', *, *, #11220, .T. ) ;
#8267=CARTESIAN_POINT ( 'NONE',  ( -7.842567732804186953, -15.33719123370038240, 38.07179725965208661 ) ) ;
#8287=ORIENTED_EDGE ( 'NONE', *, *, #41365, .T. ) ;
#8370=EDGE_CURVE ( 'NONE', #34231, #24610, #20153, .T. ) ;
#8403=LINE ( 'NONE', #5852, #22547 ) ;
#8404=EDGE_CURVE ( 'NONE', #24046, #11300, #3355, .T. ) ;
#8412=VERTEX_POINT ( 'NONE', #28876 ) ;
#8423=ORIENTED_EDGE ( 'NONE', *, *, #31455, .F. ) ;
#8431=CARTESIAN_POINT ( 'NONE',  ( 22.99999999999999645, -10.75000000000000000, -52.99999999999997868 ) ) ;
#8463=LINE ( 'NONE', #24435, #5704 ) ;
#8470=CARTESIAN_POINT ( 'NONE',  ( 4.257384923554909051, -9.749999999999998224, 29.19375250200204164 ) ) ;
#8476=VERTEX_POINT ( 'NONE', #33759 ) ;
#8482=DIRECTION ( 'NONE',  ( 0.000000000000000000, 1.000000000000000000, 0.000000000000000000 ) ) ;
#8522=ORIENTED_EDGE ( 'NONE', *, *, #6560, .T. ) ;
#8524=DIRECTION ( 'NONE',  ( 0.000000000000000000, -1.000000000000000000, 0.000000000000000000 ) ) ;
#8534=ORIENTED_EDGE ( 'NONE', *, *, #2728, .T. ) ;
#8579=DIRECTION ( 'NONE',  ( 0.000000000000000000, -1.000000000000000000, 0.000000000000000000 ) ) ;
#8594=DIRECTION ( 'NONE',  ( 0.000000000000000000, 0.000000000000000000, -1.000000000000000000 ) ) ;
#8624=VERTEX_POINT ( 'NONE', #27374 ) ;
#8629=CARTESIAN_POINT ( 'NONE',  ( 30.00000000000002487, -3.250000000000000444, -13.91584042252960529 ) ) ;
#8638=ORIENTED_EDGE ( 'NONE', *, *, #24708, .F. ) ;
#8727=CARTESIAN_POINT ( 'NONE',  ( 29.99999999999999645, -5.749999999999999112, -45.99999999999998579 ) ) ;
#8731=VERTEX_POINT ( 'NONE', #5442 ) ;
#8740=AXIS2_PLACEMENT_3D ( 'NONE', #40077, #7120, #956 ) ;
#8749=EDGE_CURVE ( 'NONE', #27946, #4073, #26054, .T. ) ;
#8785=EDGE_LOOP ( 'NONE', ( #19928, #18944, #7912, #20997 ) ) ;
#8812=DIRECTION ( 'NONE',  ( 1.000000000000000000, 0.000000000000000000, -3.672050975999536074E-16 ) ) ;
#8814=LINE ( 'NONE', #7618, #22075 ) ;
#8823=CARTESIAN_POINT ( 'NONE',  ( 30.00000000000000000, -9.749999999999998224, -18.08432671081678578 ) ) ;
#8825=CARTESIAN_POINT ( 'NONE',  ( -72.11291920797204114, -3.250000000000000444, 14.09998371085514179 ) ) ;
#8855=FACE_OUTER_BOUND ( 'NONE', #37121, .T. ) ;
#8881=CARTESIAN_POINT ( 'NONE',  ( 7.651048906156357354, 0.7499999999999997780, 14.58269351323625074 ) ) ;
#8899=ORIENTED_EDGE ( 'NONE', *, *, #25251, .F. ) ;
#8915=CARTESIAN_POINT ( 'NONE',  ( 14.23381301606215743, 0.7499999999999997780, -13.75869656311284217 ) ) ;
#8940=ORIENTED_EDGE ( 'NONE', *, *, #27495, .T. ) ;
#8948=DIRECTION ( 'NONE',  ( 3.672050975999536074E-16, -0.000000000000000000, 1.000000000000000000 ) ) ;
#8988=CARTESIAN_POINT ( 'NONE',  ( 4.257384923554909051, 7.250000000000000000, 29.19375250200204164 ) ) ;
#8994=EDGE_CURVE ( 'NONE', #41416, #39128, #6598, .T. ) ;
#9031=LINE ( 'NONE', #15429, #40984 ) ;
#9035=AXIS2_PLACEMENT_3D ( 'NONE', #14859, #30603, #4659 ) ;
#9057=ORIENTED_EDGE ( 'NONE', *, *, #13164, .T. ) ;
#9068=DIRECTION ( 'NONE',  ( 0.000000000000000000, 0.000000000000000000, -1.000000000000000000 ) ) ;
#9090=CARTESIAN_POINT ( 'NONE',  ( 30.00000000000000000, -5.749999999999998224, -13.91584042252958930 ) ) ;
#9107=CARTESIAN_POINT ( 'NONE',  ( 29.99999999999999645, -3.250000000000000444, -45.99999999999998579 ) ) ;
#9108=ORIENTED_EDGE ( 'NONE', *, *, #31341, .F. ) ;
#9119=CARTESIAN_POINT ( 'NONE',  ( 15.15956014310333622, 6.503469248131256819, 39.52179012744504405 ) ) ;
#9122=ORIENTED_EDGE ( 'NONE', *, *, #38170, .F. ) ;
#9125=AXIS2_PLACEMENT_3D ( 'NONE', #15061, #32053, #34828 ) ;
#9135=CARTESIAN_POINT ( 'NONE',  ( -8.389070150686304572, 6.164615742443255719, 37.27435362516997941 ) ) ;
#9173=ORIENTED_EDGE ( 'NONE', *, *, #11871, .T. ) ;
#9200=CARTESIAN_POINT ( 'NONE',  ( -11.21606888246744127, -9.749999999999998224, 29.19375250200204519 ) ) ;
#9207=EDGE_CURVE ( 'NONE', #41095, #41715, #34220, .T. ) ;
#9216=CARTESIAN_POINT ( 'NONE',  ( 4.257384923554909051, 7.250000000000000000, 29.19375250200204164 ) ) ;
#9222=EDGE_LOOP ( 'NONE', ( #26188, #12179, #30837, #9108 ) ) ;
#9227=AXIS2_PLACEMENT_3D ( 'NONE', #19165, #10015, #31710 ) ;
#9234=CARTESIAN_POINT ( 'NONE',  ( -26.68952268848979870, -5.749999999999999112, 29.19375250200205230 ) ) ;
#9251=CARTESIAN_POINT ( 'NONE',  ( -10.63967459768254820, 1.750000000000001554, 30.94806650488419564 ) ) ;
#9254=CARTESIAN_POINT ( 'NONE',  ( -17.89728711128011440, 1.750000000000001554, 32.19375250200205585 ) ) ;
#9277=ORIENTED_EDGE ( 'NONE', *, *, #30652, .F. ) ;
#9279=DIRECTION ( 'NONE',  ( 0.000000000000000000, 0.000000000000000000, 1.000000000000000000 ) ) ;
#9325=DIRECTION ( 'NONE',  ( 2.768405754343413644E-16, 0.000000000000000000, 1.000000000000000000 ) ) ;
#9351=CARTESIAN_POINT ( 'NONE',  ( -3.170115195858332235, 6.278445815741363845, 42.26165866505093049 ) ) ;
#9387=CARTESIAN_POINT ( 'NONE',  ( 11.02911845508759470, 0.7500000000000006661, -8.710966395423659137 ) ) ;
#9472=DIRECTION ( 'NONE',  ( 0.000000000000000000, 0.000000000000000000, -1.000000000000000000 ) ) ;
#9479=VECTOR ( 'NONE', #33156, 1000.000000000000000 ) ;
#9515=CARTESIAN_POINT ( 'NONE',  ( -2.668805347656625298E-15, -4.500000000000000000, 40.00000000000002132 ) ) ;
#9527=APPLICATION_CONTEXT ( 'automotive_design' ) ;
#9536=DIRECTION ( 'NONE',  ( 2.768405754343413644E-16, 0.000000000000000000, 1.000000000000000000 ) ) ;
#9541=ORIENTED_EDGE ( 'NONE', *, *, #8027, .T. ) ;
#9545=ORIENTED_EDGE ( 'NONE', *, *, #8370, .T. ) ;
#9580=CARTESIAN_POINT ( 'NONE',  ( 4.257384923554909051, -19.75000000000000000, 34.69375250200203453 ) ) ;
#9622=DIRECTION ( 'NONE',  ( 0.000000000000000000, 0.000000000000000000, -1.000000000000000000 ) ) ;
#9643=AXIS2_PLACEMENT_3D ( 'NONE', #40421, #16827, #11281 ) ;
#9649=CARTESIAN_POINT ( 'NONE',  ( 22.99999999999999645, -10.75000000000000000, -55.99999999999998579 ) ) ;
#9691=CARTESIAN_POINT ( 'NONE',  ( 30.00000000000000711, 0.7500000000000002220, -13.91584042252959286 ) ) ;
#9705=ORIENTED_EDGE ( 'NONE', *, *, #11220, .F. ) ;
#9708=DIRECTION ( 'NONE',  ( 0.000000000000000000, 0.000000000000000000, -1.000000000000000000 ) ) ;
#9714=LINE ( 'NONE', #35653, #33926 ) ;
#9745=CARTESIAN_POINT ( 'NONE',  ( -91.72768752788732627, -3.250000000000000444, -57.39251435732919049 ) ) ;
#9756=ADVANCED_FACE ( 'NONE', ( #6882 ), #16681, .T. ) ;
#9768=CARTESIAN_POINT ( 'NONE',  ( 17.89728711128010730, -4.500000000000000000, 40.00000000000002842 ) ) ;
#9785=CARTESIAN_POINT ( 'NONE',  ( 1.830729938757765352, 5.745867447553131946, 44.00401676599550171 ) ) ;
#9795=FACE_OUTER_BOUND ( 'NONE', #18797, .T. ) ;
#9800=FACE_OUTER_BOUND ( 'NONE', #28618, .T. ) ;
#9817=AXIS2_PLACEMENT_3D ( 'NONE', #38400, #38607, #9472 ) ;
#9872=EDGE_CURVE ( 'NONE', #38940, #39544, #4954, .T. ) ;
#9890=LINE ( 'NONE', #19240, #24032 ) ;
#9905=CYLINDRICAL_SURFACE ( 'NONE', #37507, 9.999999999999980460 ) ;
#9924=ORIENTED_EDGE ( 'NONE', *, *, #8027, .F. ) ;
#9970=ORIENTED_EDGE ( 'NONE', *, *, #14513, .T. ) ;
#10015=DIRECTION ( 'NONE',  ( -0.000000000000000000, -1.000000000000000000, -0.000000000000000000 ) ) ;
#10030=CARTESIAN_POINT ( 'NONE',  ( 4.257384923554909051, -19.75000000000000000, 29.19375250200204164 ) ) ;
#10033=CARTESIAN_POINT ( 'NONE',  ( -26.68952268848979870, 1.749999999999999778, 29.19375250200205230 ) ) ;
#10048=PLANE ( 'NONE',  #29870 ) ;
#10088=EDGE_CURVE ( 'NONE', #28670, #15662, #13078, .T. ) ;
#10096=ORIENTED_EDGE ( 'NONE', *, *, #17298, .T. ) ;
#10109=EDGE_LOOP ( 'NONE', ( #39781, #28137, #33273, #36790 ) ) ;
#10115=CARTESIAN_POINT ( 'NONE',  ( -33.00000000000002132, -4.500000000000000000, 40.00000000000001421 ) ) ;
#10172=ADVANCED_FACE ( 'NONE', ( #32773 ), #19804, .F. ) ;
#10173=DIRECTION ( 'NONE',  ( 0.000000000000000000, 0.000000000000000000, -1.000000000000000000 ) ) ;
#10211=ORIENTED_EDGE ( 'NONE', *, *, #24448, .T. ) ;
#10221=ORIENTED_EDGE ( 'NONE', *, *, #29057, .F. ) ;
#10249=ORIENTED_EDGE ( 'NONE', *, *, #16821, .T. ) ;
#10300=ORIENTED_EDGE ( 'NONE', *, *, #8080, .F. ) ;
#10304=CARTESIAN_POINT ( 'NONE',  ( -91.72768752788732627, -5.749999999999999112, -57.39251435732919049 ) ) ;
#10317=ORIENTED_EDGE ( 'NONE', *, *, #4553, .T. ) ;
#10401=CARTESIAN_POINT ( 'NONE',  ( 17.61740008252201406, -14.78703941992704962, 36.04667029275037748 ) ) ;
#10420=ORIENTED_EDGE ( 'NONE', *, *, #40650, .F. ) ;
#10447=CARTESIAN_POINT ( 'NONE',  ( 22.99999999999999645, 1.750000000000001554, -45.99999999999998579 ) ) ;
#10474=ORIENTED_EDGE ( 'NONE', *, *, #29492, .F. ) ;
#10487=AXIS2_PLACEMENT_3D ( 'NONE', #15056, #32048, #6315 ) ;
#10488=SHAPE_REPRESENTATION_RELATIONSHIP ( 'NONE' , 'NONE' ,  #32103, #29470 ) ;
#10514=EDGE_LOOP ( 'NONE', ( #5134, #30870 ) ) ;
#10562=DIRECTION ( 'NONE',  ( 0.000000000000000000, 0.000000000000000000, -1.000000000000000000 ) ) ;
#10614=CARTESIAN_POINT ( 'NONE',  ( 10.19014111864197325, -15.09110772812408818, 42.97531106287303260 ) ) ;
#10641=ORIENTED_EDGE ( 'NONE', *, *, #3221, .T. ) ;
#10720=ORIENTED_EDGE ( 'NONE', *, *, #905, .T. ) ;
#10737=ORIENTED_EDGE ( 'NONE', *, *, #28577, .F. ) ;
#10739=CARTESIAN_POINT ( 'NONE',  ( 18.95432338025397456, -10.75000000000000000, 32.19375250200202743 ) ) ;
#10775=EDGE_LOOP ( 'NONE', ( #8534, #14231, #36532, #32182 ) ) ;
#10786=VECTOR ( 'NONE', #579, 1000.000000000000000 ) ;
#10799=ADVANCED_FACE ( 'NONE', ( #30813 ), #21238, .T. ) ;
#10816=ADVANCED_FACE ( 'NONE', ( #40591 ), #30181, .F. ) ;
#10820=ADVANCED_FACE ( 'NONE', ( #1877 ), #40799, .F. ) ;
#10892=VECTOR ( 'NONE', #10173, 1000.000000000000000 ) ;
#10894=LINE ( 'NONE', #23664, #26490 ) ;
#10895=CARTESIAN_POINT ( 'NONE',  ( 29.99999999999999645, -3.250000000000000444, -45.99999999999998579 ) ) ;
#10955=CARTESIAN_POINT ( 'NONE',  ( 18.86175345918892177, -11.31641900065896600, 32.64725064628024853 ) ) ;
#10958=ORIENTED_EDGE ( 'NONE', *, *, #14639, .T. ) ;
#11003=EDGE_LOOP ( 'NONE', ( #25227, #15488, #19168 ) ) ;
#11009=ORIENTED_EDGE ( 'NONE', *, *, #20144, .F. ) ;
#11014=DIRECTION ( 'NONE',  ( -0.000000000000000000, 1.000000000000000000, -0.000000000000000000 ) ) ;
#11038=CARTESIAN_POINT ( 'NONE',  ( 30.00000000000001776, -5.749999999999999112, 29.19375250200203098 ) ) ;
#11050=DIRECTION ( 'NONE',  ( -3.469446951953623557E-16, 0.000000000000000000, 1.000000000000000000 ) ) ;
#11061=VECTOR ( 'NONE', #33717, 1000.000000000000000 ) ;
#11131=CARTESIAN_POINT ( 'NONE',  ( 0.000000000000000000, 0.000000000000000000, 0.000000000000000000 ) ) ;
#11154=AXIS2_PLACEMENT_3D ( 'NONE', #35471, #21648, #6118 ) ;
#11217=VERTEX_POINT ( 'NONE', #37031 ) ;
#11220=EDGE_CURVE ( 'NONE', #32144, #27293, #33406, .T. ) ;
#11223=FACE_OUTER_BOUND ( 'NONE', #24310, .T. ) ;
#11227=CARTESIAN_POINT ( 'NONE',  ( 23.34627465269464253, -3.250000000000000444, -52.99143003003683816 ) ) ;
#11237=CYLINDRICAL_SURFACE ( 'NONE', #19792, 105.2919410404669378 ) ;
#11254=CARTESIAN_POINT ( 'NONE',  ( -8.632135858800516814, -15.05720047843595921, 36.88015005047475370 ) ) ;
#11281=DIRECTION ( 'NONE',  ( 0.000000000000000000, -0.000000000000000000, -1.000000000000000000 ) ) ;
#11291=DIRECTION ( 'NONE',  ( 0.000000000000000000, 0.000000000000000000, -1.000000000000000000 ) ) ;
#11295=DIRECTION ( 'NONE',  ( 0.000000000000000000, -0.000000000000000000, -1.000000000000000000 ) ) ;
#11300=VERTEX_POINT ( 'NONE', #30215 ) ;
#11303=DIRECTION ( 'NONE',  ( 0.000000000000000000, 1.000000000000000000, 0.000000000000000000 ) ) ;
#11308=VERTEX_POINT ( 'NONE', #19496 ) ;
#11311=CARTESIAN_POINT ( 'NONE',  ( 30.00000000000000000, 21.91020392607983780, -18.08432671081678578 ) ) ;
#11351=ADVANCED_FACE ( 'NONE', ( #16319 ), #12909, .F. ) ;
#11362=ORIENTED_EDGE ( 'NONE', *, *, #21660, .F. ) ;
#11371=PLANE ( 'NONE',  #4811 ) ;
#11408=ORIENTED_EDGE ( 'NONE', *, *, #30097, .F. ) ;
#11415=ORIENTED_EDGE ( 'NONE', *, *, #30634, .T. ) ;
#11450=DIRECTION ( 'NONE',  ( 0.000000000000000000, 0.000000000000000000, -1.000000000000000000 ) ) ;
#11455=CARTESIAN_POINT ( 'NONE',  ( 4.257384923554909051, 0.7499999999999997780, 14.19375250200204341 ) ) ;
#11461=ORIENTED_EDGE ( 'NONE', *, *, #36859, .T. ) ;
#11509=LINE ( 'NONE', #21096, #23883 ) ;
#11575=EDGE_CURVE ( 'NONE', #41673, #32751, #33088, .T. ) ;
#11587=DIRECTION ( 'NONE',  ( 0.2645837230171118049, -0.000000000000000000, 0.9643627188534428241 ) ) ;
#11599=ORIENTED_EDGE ( 'NONE', *, *, #16818, .F. ) ;
#11613=EDGE_CURVE ( 'NONE', #31717, #7396, #7361, .T. ) ;
#11655=CARTESIAN_POINT ( 'NONE',  ( 4.257384923554910827, -14.66919072256743561, 44.19375250200204164 ) ) ;
#11669=ADVANCED_FACE ( 'NONE', ( #36928 ), #36070, .F. ) ;
#11722=ORIENTED_EDGE ( 'NONE', *, *, #2728, .F. ) ;
#11765=VECTOR ( 'NONE', #35401, 1000.000000000000000 ) ;
#11778=DIRECTION ( 'NONE',  ( 0.000000000000000000, 0.000000000000000000, 1.000000000000000000 ) ) ;
#11806=EDGE_CURVE ( 'NONE', #16080, #29045, #34865, .T. ) ;
#11816=PLANE ( 'NONE',  #26641 ) ;
#11846=AXIS2_PLACEMENT_3D ( 'NONE', #31420, #15906, #28853 ) ;
#11861=CIRCLE ( 'NONE', #23445, 6.999999999999992006 ) ;
#11862=VERTEX_POINT ( 'NONE', #37964 ) ;
#11871=EDGE_CURVE ( 'NONE', #21343, #23286, #40946, .T. ) ;
#11880=ORIENTED_EDGE ( 'NONE', *, *, #14043, .F. ) ;
#11919=CARTESIAN_POINT ( 'NONE',  ( 7.651048906156353802, 7.250000000000000000, 14.58269351323625251 ) ) ;
#11929=DIRECTION ( 'NONE',  ( 0.08163352362547933450, 0.000000000000000000, 0.9966624141706600382 ) ) ;
#11966=ADVANCED_FACE ( 'NONE', ( #21586 ), #30960, .F. ) ;
#11975=LINE ( 'NONE', #34734, #33175 ) ;
#11977=CARTESIAN_POINT ( 'NONE',  ( 4.257384923554909051, 1.750000000000001554, 29.19375250200204164 ) ) ;
#11986=EDGE_LOOP ( 'NONE', ( #437, #25029 ) ) ;
#11993=EDGE_CURVE ( 'NONE', #35361, #12679, #2864, .T. ) ;
#12008=CYLINDRICAL_SURFACE ( 'NONE', #27517, 10.99999999999998934 ) ;
#12046=DIRECTION ( 'NONE',  ( 1.000000000000000000, 0.000000000000000000, 2.102695122396128930E-16 ) ) ;
#12090=CARTESIAN_POINT ( 'NONE',  ( 17.27288510725846393, 5.985041993372042235, 36.65812737060138460 ) ) ;
#12103=PLANE ( 'NONE',  #22060 ) ;
#12133=PLANE ( 'NONE',  #18430 ) ;
#12137=EDGE_CURVE ( 'NONE', #33277, #13653, #9890, .T. ) ;
#12147=EDGE_CURVE ( 'NONE', #12570, #37363, #9031, .T. ) ;
#12164=AXIS2_PLACEMENT_3D ( 'NONE', #35310, #22965, #16599 ) ;
#12179=ORIENTED_EDGE ( 'NONE', *, *, #534, .F. ) ;
#12200=CARTESIAN_POINT ( 'NONE',  ( 4.257384923554909051, 0.7499999999999997780, 29.19375250200204164 ) ) ;
#12242=VECTOR ( 'NONE', #40147, 1000.000000000000000 ) ;
#12249=VERTEX_POINT ( 'NONE', #33895 ) ;
#12308=CARTESIAN_POINT ( 'NONE',  ( 4.976604849439111966, 5.669190722567437390, 44.19375250200205585 ) ) ;
#12353=ADVANCED_FACE ( 'NONE', ( #9795 ), #35728, .T. ) ;
#12396=ORIENTED_EDGE ( 'NONE', *, *, #25589, .T. ) ;
#12413=ORIENTED_EDGE ( 'NONE', *, *, #14353, .F. ) ;
#12469=CARTESIAN_POINT ( 'NONE',  ( 4.257384923554909051, 0.7499999999999997780, 29.19375250200204164 ) ) ;
#12476=LINE ( 'NONE', #19066, #8119 ) ;
#12493=CARTESIAN_POINT ( 'NONE',  ( 22.99999999999999645, 1.750000000000001554, -55.99999999999998579 ) ) ;
#12496=DIRECTION ( 'NONE',  ( -0.000000000000000000, -1.000000000000000000, -0.000000000000000000 ) ) ;
#12509=CARTESIAN_POINT ( 'NONE',  ( -10.63967459768254642, -10.75000000000000000, 30.94806650488419564 ) ) ;
#12526=CARTESIAN_POINT ( 'NONE',  ( 7.103374011260529919, 5.775982313707774374, 43.92566714239928416 ) ) ;
#12533=LINE ( 'NONE', #8915, #15267 ) ;
#12539=CARTESIAN_POINT ( 'NONE',  ( -10.18284942939592241, 4.195061311404153059, 33.25815295540223815 ) ) ;
#12553=DIRECTION ( 'NONE',  ( -2.102695122396128190E-16, 0.000000000000000000, 1.000000000000000000 ) ) ;
#12564=ORIENTED_EDGE ( 'NONE', *, *, #29628, .T. ) ;
#12570=VERTEX_POINT ( 'NONE', #24653 ) ;
#12575=DIRECTION ( 'NONE',  ( 0.9643627188534427130, 0.000000000000000000, -0.2645837230171119159 ) ) ;
#12605=DIRECTION ( 'NONE',  ( 0.000000000000000000, -1.000000000000000000, 0.000000000000000000 ) ) ;
#12612=CARTESIAN_POINT ( 'NONE',  ( -12.28065031820330155, -9.749999999999998224, 16.19629439043522012 ) ) ;
#12617=EDGE_CURVE ( 'NONE', #5713, #27293, #3539, .T. ) ;
#12620=EDGE_CURVE ( 'NONE', #33817, #26221, #21711, .T. ) ;
#12679=VERTEX_POINT ( 'NONE', #5916 ) ;
#12680=VERTEX_POINT ( 'NONE', #16339 ) ;
#12699=EDGE_CURVE ( 'NONE', #35877, #42083, #18886, .T. ) ;
#12767=FACE_OUTER_BOUND ( 'NONE', #17126, .T. ) ;
#12781=ORIENTED_EDGE ( 'NONE', *, *, #338, .F. ) ;
#12786=ORIENTED_EDGE ( 'NONE', *, *, #732, .F. ) ;
#12812=DIRECTION ( 'NONE',  ( -0.000000000000000000, 1.000000000000000000, -0.000000000000000000 ) ) ;
#12814=CIRCLE ( 'NONE', #2611, 9.999999999999980460 ) ;
#12849=LINE ( 'NONE', #15847, #2124 ) ;
#12874=CARTESIAN_POINT ( 'NONE',  ( -2.668805347656625298E-15, -4.500000000000000000, 40.00000000000002132 ) ) ;
#12893=LINE ( 'NONE', #6512, #738 ) ;
#12906=AXIS2_PLACEMENT_3D ( 'NONE', #15071, #31026, #28034 ) ;
#12909=PLANE ( 'NONE',  #39603 ) ;
#12925=EDGE_CURVE ( 'NONE', #33538, #35318, #21348, .T. ) ;
#12949=CARTESIAN_POINT ( 'NONE',  ( 11.15595245335247299, 6.208956458674490975, 42.53232886660664747 ) ) ;
#12986=CARTESIAN_POINT ( 'NONE',  ( 18.95432338025397812, 1.750000000000001554, 32.19375250200202743 ) ) ;
#12993=CARTESIAN_POINT ( 'NONE',  ( 23.34627465269464253, -9.749999999999998224, -52.99143003003683816 ) ) ;
#13003=VECTOR ( 'NONE', #40998, 1000.000000000000114 ) ;
#13017=CARTESIAN_POINT ( 'NONE',  ( 4.257384923554909051, 7.250000000000000000, 29.19375250200204164 ) ) ;
#13044=VECTOR ( 'NONE', #9536, 1000.000000000000000 ) ;
#13078=CIRCLE ( 'NONE', #41598, 108.2919410404669378 ) ;
#13130=EDGE_CURVE ( 'NONE', #11862, #12249, #15791, .T. ) ;
#13142=CARTESIAN_POINT ( 'NONE',  ( -26.68952268848979870, -3.250000000000000444, 29.19375250200205230 ) ) ;
#13143=VECTOR ( 'NONE', #16527, 1000.000000000000000 ) ;
#13164=EDGE_CURVE ( 'NONE', #5338, #28829, #3874, .T. ) ;
#13165=CARTESIAN_POINT ( 'NONE',  ( 11.16916954227777481, -15.21058235723968366, 42.52578322251227405 ) ) ;
#13179=CARTESIAN_POINT ( 'NONE',  ( -2.668805347656625298E-15, -4.500000000000000000, 40.00000000000002132 ) ) ;
#13187=DIRECTION ( 'NONE',  ( -0.000000000000000000, -1.000000000000000000, -0.000000000000000000 ) ) ;
#13195=DIRECTION ( 'NONE',  ( -1.000000000000000000, -0.000000000000000000, -2.102695122396128930E-16 ) ) ;
#13197=EDGE_CURVE ( 'NONE', #223, #26221, #8403, .T. ) ;
#13200=AXIS2_PLACEMENT_3D ( 'NONE', #24959, #3434, #25789 ) ;
#13230=DIRECTION ( 'NONE',  ( -0.000000000000000000, -1.000000000000000000, -0.000000000000000000 ) ) ;
#13232=VERTEX_POINT ( 'NONE', #9251 ) ;
#13244=ORIENTED_EDGE ( 'NONE', *, *, #39172, .F. ) ;
#13259=PRODUCT_DEFINITION_FORMATION_WITH_SPECIFIED_SOURCE ( 'ANY', '', #21777, .NOT_KNOWN. ) ;
#13260=VECTOR ( 'NONE', #18976, 1000.000000000000000 ) ;
#13290=B_SPLINE_CURVE_WITH_KNOTS ( 'NONE', 3,
 ( #25510, #12308, #28263, #15310, #12526, #38256, #22510, #25717, #25928, #12949, #35071, #38474, #5931, #31453, #9119, #41247, #6140, #22099, #12090, #42095, #3166, #31870 ),
 .UNSPECIFIED., .F., .F.,
 ( 4, 2, 2, 2, 2, 2, 2, 2, 2, 2, 4 ),
 ( 0.02327094513562554326, 0.02542445434304105994, 0.02650120894674882002, 0.02757796355045658010, 0.02973147275787210719, 0.03188498196528764123, 0.03403849117270316832, 0.03619200038011870235, 0.03834550958753422945, 0.03942226419124200687, 0.04049901879494977736 ),
 .UNSPECIFIED. ) ;
#13311=DIRECTION ( 'NONE',  ( -0.000000000000000000, -1.000000000000000000, -0.000000000000000000 ) ) ;
#13350=DIRECTION ( 'NONE',  ( 0.000000000000000000, -1.000000000000000000, 0.000000000000000000 ) ) ;
#13431=CARTESIAN_POINT ( 'NONE',  ( 22.99999999999999645, 1.750000000000001554, -55.99999999999998579 ) ) ;
#13500=VERTEX_POINT ( 'NONE', #32828 ) ;
#13570=AXIS2_PLACEMENT_3D ( 'NONE', #25704, #19727, #28878 ) ;
#13581=CARTESIAN_POINT ( 'NONE',  ( -33.00000000000002842, -4.500000000000000000, 40.00000000000001421 ) ) ;
#13609=EDGE_CURVE ( 'NONE', #36201, #30663, #42011, .T. ) ;
#13653=VERTEX_POINT ( 'NONE', #8431 ) ;
#13668=DIRECTION ( 'NONE',  ( -0.000000000000000000, -1.000000000000000000, -0.000000000000000000 ) ) ;
#13694=DIRECTION ( 'NONE',  ( 0.9740705992510528821, -0.000000000000000000, 0.2262442655067633257 ) ) ;
#13723=ORIENTED_EDGE ( 'NONE', *, *, #22335, .F. ) ;
#13729=( NAMED_UNIT ( * ) PLANE_ANGLE_UNIT ( ) SI_UNIT ( $, .RADIAN. ) );
#13787=AXIS2_PLACEMENT_3D ( 'NONE', #14981, #34540, #8594 ) ;
#13801=ADVANCED_FACE ( 'NONE', ( #11223 ), #27385, .T. ) ;
#13802=CARTESIAN_POINT ( 'NONE',  ( 15.17249539544035919, -15.50266705007750723, 39.50773913691367056 ) ) ;
#13814=AXIS2_PLACEMENT_3D ( 'NONE', #27760, #11587, #84 ) ;
#13819=CIRCLE ( 'NONE', #24684, 10.00000000000000178 ) ;
#13903=AXIS2_PLACEMENT_3D ( 'NONE', #33672, #23239, #4524 ) ;
#13932=CARTESIAN_POINT ( 'NONE',  ( 29.99999999999999645, -10.75000000000000000, -45.99999999999998579 ) ) ;
#13933=CIRCLE ( 'NONE', #32927, 14.99999999999999822 ) ;
#13984=ADVANCED_FACE ( 'NONE', ( #8855 ), #21829, .T. ) ;
#13992=VECTOR ( 'NONE', #15391, 1000.000000000000000 ) ;
#14016=DIRECTION ( 'NONE',  ( -0.000000000000000000, -1.000000000000000000, -0.000000000000000000 ) ) ;
#14043=EDGE_CURVE ( 'NONE', #24819, #33170, #21253, .T. ) ;
#14084=ORIENTED_EDGE ( 'NONE', *, *, #21470, .T. ) ;
#14086=CARTESIAN_POINT ( 'NONE',  ( 17.89728711128010730, 7.250000000000000000, 35.43499182679077109 ) ) ;
#14088=ORIENTED_EDGE ( 'NONE', *, *, #24119, .T. ) ;
#14097=ORIENTED_EDGE ( 'NONE', *, *, #25612, .T. ) ;
#14146=ORIENTED_EDGE ( 'NONE', *, *, #41365, .F. ) ;
#14150=EDGE_CURVE ( 'NONE', #8476, #41416, #17158, .T. ) ;
#14214=VECTOR ( 'NONE', #38035, 1000.000000000000000 ) ;
#14220=CARTESIAN_POINT ( 'NONE',  ( -26.68952268848979870, -10.75000000000000000, 29.19375250200205230 ) ) ;
#14231=ORIENTED_EDGE ( 'NONE', *, *, #20427, .T. ) ;
#14234=CARTESIAN_POINT ( 'NONE',  ( 22.99999999999999645, -5.749999999999999112, -45.99999999999998579 ) ) ;
#14251=VECTOR ( 'NONE', #2921, 1000.000000000000000 ) ;
#14255=VECTOR ( 'NONE', #17694, 1000.000000000000000 ) ;
#14257=VERTEX_POINT ( 'NONE', #22452 ) ;
#14258=CARTESIAN_POINT ( 'NONE',  ( 4.257384923554909051, -19.75000000000000000, 29.19375250200204164 ) ) ;
#14270=DIRECTION ( 'NONE',  ( 0.000000000000000000, -1.000000000000000000, 0.000000000000000000 ) ) ;
#14273=VECTOR ( 'NONE', #1361, 1000.000000000000114 ) ;
#14305=VECTOR ( 'NONE', #3287, 1000.000000000000000 ) ;
#14338=CIRCLE ( 'NONE', #1399, 108.2919410404669378 ) ;
#14341=FACE_OUTER_BOUND ( 'NONE', #31589, .T. ) ;
#14353=EDGE_CURVE ( 'NONE', #11217, #29182, #14569, .T. ) ;
#14365=LINE ( 'NONE', #30736, #6754 ) ;
#14378=DIRECTION ( 'NONE',  ( -1.000000000000000000, -0.000000000000000000, -2.102695122396128930E-16 ) ) ;
#14403=ORIENTED_EDGE ( 'NONE', *, *, #16154, .F. ) ;
#14422=VECTOR ( 'NONE', #36795, 1000.000000000000000 ) ;
#14449=CARTESIAN_POINT ( 'NONE',  ( -7.550624573573786691, -15.39778602303815092, 38.45713824087260946 ) ) ;
#14456=ORIENTED_EDGE ( 'NONE', *, *, #36682, .F. ) ;
#14467=DIRECTION ( 'NONE',  ( 0.000000000000000000, 0.000000000000000000, -1.000000000000000000 ) ) ;
#14507=ORIENTED_EDGE ( 'NONE', *, *, #7735, .F. ) ;
#14511=ORIENTED_EDGE ( 'NONE', *, *, #41434, .F. ) ;
#14513=EDGE_CURVE ( 'NONE', #33277, #39224, #1549, .T. ) ;
#14517=ADVANCED_FACE ( 'NONE', ( #41348 ), #15615, .T. ) ;
#14569=LINE ( 'NONE', #13932, #11061 ) ;
#14578=DIRECTION ( 'NONE',  ( 0.000000000000000000, 0.000000000000000000, -1.000000000000000000 ) ) ;
#14616=VERTEX_POINT ( 'NONE', #9649 ) ;
#14639=EDGE_CURVE ( 'NONE', #569, #30721, #19215, .T. ) ;
#14643=CIRCLE ( 'NONE', #20783, 15.00000000000000000 ) ;
#14671=EDGE_CURVE ( 'NONE', #41490, #5338, #35589, .T. ) ;
#14691=DIRECTION ( 'NONE',  ( 1.000000000000000000, 0.000000000000000000, 2.102695122396128930E-16 ) ) ;
#14711=CARTESIAN_POINT ( 'NONE',  ( 23.34627465269464253, 0.7499999999999997780, -52.99143003003683816 ) ) ;
#14715=DIRECTION ( 'NONE',  ( 1.000000000000000000, 0.000000000000000000, 2.102695122396128930E-16 ) ) ;
#14723=DIRECTION ( 'NONE',  ( -0.08163352362547934837, -0.000000000000000000, -0.9966624141706601492 ) ) ;
#14730=DIRECTION ( 'NONE',  ( 0.000000000000000000, 0.000000000000000000, -1.000000000000000000 ) ) ;
#14753=DIRECTION ( 'NONE',  ( 0.000000000000000000, 1.000000000000000000, 0.000000000000000000 ) ) ;
#14766=CYLINDRICAL_SURFACE ( 'NONE', #15619, 14.99999999999999822 ) ;
#14776=ORIENTED_EDGE ( 'NONE', *, *, #12620, .F. ) ;
#14794=DIRECTION ( 'NONE',  ( -0.000000000000000000, 1.000000000000000000, -0.000000000000000000 ) ) ;
#14797=CARTESIAN_POINT ( 'NONE',  ( -33.00000000000001421, -10.75000000000000000, 30.00000000000003908 ) ) ;
#14824=ORIENTED_EDGE ( 'NONE', *, *, #30369, .T. ) ;
#14825=ORIENTED_EDGE ( 'NONE', *, *, #40486, .F. ) ;
#14859=CARTESIAN_POINT ( 'NONE',  ( 11.02911845508759470, 21.91020392607983780, -8.710966395423659137 ) ) ;
#14866=DIRECTION ( 'NONE',  ( 0.000000000000000000, -1.000000000000000000, 0.000000000000000000 ) ) ;
#14870=CARTESIAN_POINT ( 'NONE',  ( -73.17652798666306069, -5.749999999999999112, 10.22331041471092483 ) ) ;
#14881=MECHANICAL_DESIGN_GEOMETRIC_PRESENTATION_REPRESENTATION('',(#22384),#1980);
#14908=ORIENTED_EDGE ( 'NONE', *, *, #27724, .F. ) ;
#14916=ORIENTED_EDGE ( 'NONE', *, *, #29531, .F. ) ;
#14948=CARTESIAN_POINT ( 'NONE',  ( -17.89728711128011795, -4.500000000000000000, 49.99999999999998579 ) ) ;
#14981=CARTESIAN_POINT ( 'NONE',  ( 22.99999999999999645, -9.749999999999998224, -45.99999999999998579 ) ) ;
#15018=CARTESIAN_POINT ( 'NONE',  ( 30.00000000000001776, -10.75000000000000000, 29.19375250200203098 ) ) ;
#15056=CARTESIAN_POINT ( 'NONE',  ( -17.89728711128011440, -4.500000000000000000, 40.00000000000001421 ) ) ;
#15061=CARTESIAN_POINT ( 'NONE',  ( 22.99999999999999645, -5.749999999999999112, -45.99999999999998579 ) ) ;
#15071=CARTESIAN_POINT ( 'NONE',  ( 4.257384923554909051, 7.250000000000000000, 29.19375250200204164 ) ) ;
#15072=CARTESIAN_POINT ( 'NONE',  ( -2.305270100321474835, -15.16609042655300499, 42.71636193101476664 ) ) ;
#15075=DIRECTION ( 'NONE',  ( -3.154042683594197586E-16, 0.000000000000000000, 1.000000000000000000 ) ) ;
#15087=AXIS2_PLACEMENT_3D ( 'NONE', #13179, #31686, #2556 ) ;
#15090=ORIENTED_EDGE ( 'NONE', *, *, #30634, .F. ) ;
#15132=CARTESIAN_POINT ( 'NONE',  ( 13.19971406886381970, 0.7500000000000006661, -9.306493635776057261 ) ) ;
#15142=LINE ( 'NONE', #27692, #3359 ) ;
#15175=AXIS2_PLACEMENT_3D ( 'NONE', #25588, #12812, #41541 ) ;
#15215=CIRCLE ( 'NONE', #26793, 10.00000000000000178 ) ;
#15216=DIRECTION ( 'NONE',  ( 1.178372492411205818E-15, 0.000000000000000000, 1.000000000000000000 ) ) ;
#15235=DIRECTION ( 'NONE',  ( -0.000000000000000000, -1.000000000000000000, -0.000000000000000000 ) ) ;
#15240=AXIS2_PLACEMENT_3D ( 'NONE', #34058, #17895, #31274 ) ;
#15246=EDGE_CURVE ( 'NONE', #35066, #14616, #13819, .T. ) ;
#15259=LINE ( 'NONE', #34809, #5382 ) ;
#15267=VECTOR ( 'NONE', #38483, 1000.000000000000000 ) ;
#15310=CARTESIAN_POINT ( 'NONE',  ( 6.751076020744448236, 5.751254453160042246, 43.98933419080296403 ) ) ;
#15329=ADVANCED_FACE ( 'NONE', ( #19372 ), #18954, .F. ) ;
#15366=ORIENTED_EDGE ( 'NONE', *, *, #19516, .F. ) ;
#15391=DIRECTION ( 'NONE',  ( -1.000000000000000000, 0.000000000000000000, 2.242192981248496244E-16 ) ) ;
#15397=DIRECTION ( 'NONE',  ( -0.2262442655067632979, 0.000000000000000000, 0.9740705992510528821 ) ) ;
#15400=ADVANCED_FACE ( 'NONE', ( #32543 ), #31918, .F. ) ;
#15405=ORIENTED_EDGE ( 'NONE', *, *, #12137, .F. ) ;
#15429=CARTESIAN_POINT ( 'NONE',  ( -26.68952268848979870, -5.749999999999999112, 29.19375250200205230 ) ) ;
#15441=ORIENTED_EDGE ( 'NONE', *, *, #8231, .T. ) ;
#15465=ORIENTED_EDGE ( 'NONE', *, *, #25589, .F. ) ;
#15487=CARTESIAN_POINT ( 'NONE',  ( 4.257384923554909051, 1.750000000000001554, 29.19375250200204164 ) ) ;
#15488=ORIENTED_EDGE ( 'NONE', *, *, #29181, .F. ) ;
#15556=AXIS2_PLACEMENT_3D ( 'NONE', #33761, #13350, #36955 ) ;
#15560=ORIENTED_EDGE ( 'NONE', *, *, #4957, .F. ) ;
#15567=DIRECTION ( 'NONE',  ( -0.000000000000000000, -1.000000000000000000, -0.000000000000000000 ) ) ;
#15615=PLANE ( 'NONE',  #6981 ) ;
#15619=AXIS2_PLACEMENT_3D ( 'NONE', #17531, #34319, #27529 ) ;
#15659=CARTESIAN_POINT ( 'NONE',  ( -10.74261507644508740, -9.749999999999998224, 29.19375250200204519 ) ) ;
#15662=VERTEX_POINT ( 'NONE', #27637 ) ;
#15664=VERTEX_POINT ( 'NONE', #41033 ) ;
#15669=CARTESIAN_POINT ( 'NONE',  ( -2.668805347656625298E-15, -4.500000000000000000, 40.00000000000002132 ) ) ;
#15685=UNCERTAINTY_MEASURE_WITH_UNIT (LENGTH_MEASURE( 1.000000000000000082E-05 ), #33026, 'distance_accuracy_value', 'NONE');
#15706=CARTESIAN_POINT ( 'NONE',  ( 30.00000000000000000, 0.7500000000000006661, -18.08432671081678578 ) ) ;
#15754=VERTEX_POINT ( 'NONE', #24456 ) ;
#15761=EDGE_LOOP ( 'NONE', ( #22397, #12564, #31397, #2612, #4352, #8899 ) ) ;
#15778=ORIENTED_EDGE ( 'NONE', *, *, #27724, .T. ) ;
#15791=CIRCLE ( 'NONE', #7622, 5.499999999999991118 ) ;
#15828=AXIS2_PLACEMENT_3D ( 'NONE', #15669, #38201, #34802 ) ;
#15831=DIRECTION ( 'NONE',  ( 0.000000000000000000, 0.000000000000000000, 1.000000000000000000 ) ) ;
#15847=CARTESIAN_POINT ( 'NONE',  ( -12.28065031820330155, 0.7499999999999997780, 16.19629439043522012 ) ) ;
#15854=CARTESIAN_POINT ( 'NONE',  ( -26.68952268848979870, -3.250000000000000444, 29.19375250200205230 ) ) ;
#15870=DIRECTION ( 'NONE',  ( 0.000000000000000000, 0.000000000000000000, -1.000000000000000000 ) ) ;
#15895=AXIS2_PLACEMENT_3D ( 'NONE', #29238, #38831, #9708 ) ;
#15905=DIRECTION ( 'NONE',  ( -3.469446951953618626E-16, 0.000000000000000000, 1.000000000000000000 ) ) ;
#15906=DIRECTION ( 'NONE',  ( -1.000000000000000000, -0.000000000000000000, -2.102695122396128930E-16 ) ) ;
#15911=CARTESIAN_POINT ( 'NONE',  ( -17.89728711128011795, -4.500000000000000000, 49.99999999999998579 ) ) ;
#15920=VECTOR ( 'NONE', #8524, 1000.000000000000000 ) ;
#15924=CARTESIAN_POINT ( 'NONE',  ( -10.57394493373416822, -11.55838076685107474, 31.50622126768103826 ) ) ;
#15932=AXIS2_PLACEMENT_3D ( 'NONE', #20296, #33264, #4128 ) ;
#15958=CARTESIAN_POINT ( 'NONE',  ( -5.903808337928534655, 6.502685752775146710, 40.23850025888122417 ) ) ;
#15968=EDGE_CURVE ( 'NONE', #32751, #8624, #34182, .T. ) ;
#15975=ORIENTED_EDGE ( 'NONE', *, *, #13197, .F. ) ;
#15992=DIRECTION ( 'NONE',  ( -0.9740705992510528821, 0.000000000000000000, -0.2262442655067633257 ) ) ;
#15994=ADVANCED_FACE ( 'NONE', ( #28890 ), #22935, .T. ) ;
#16010=( GEOMETRIC_REPRESENTATION_CONTEXT ( 3 ) GLOBAL_UNCERTAINTY_ASSIGNED_CONTEXT ( ( #15685 ) ) GLOBAL_UNIT_ASSIGNED_CONTEXT ( ( #33026, #27080, #16873 ) ) REPRESENTATION_CONTEXT ( 'NONE', 'WORKASPACE' ) );
#16022=DIRECTION ( 'NONE',  ( 2.768405754343413644E-16, 0.000000000000000000, 1.000000000000000000 ) ) ;
#16034=VECTOR ( 'NONE', #27925, 1000.000000000000000 ) ;
#16063=DIRECTION ( 'NONE',  ( -0.000000000000000000, -1.000000000000000000, -0.000000000000000000 ) ) ;
#16073=CARTESIAN_POINT ( 'NONE',  ( 32.99999999999999289, 1.750000000000001554, -45.99999999999999289 ) ) ;
#16080=VERTEX_POINT ( 'NONE', #19323 ) ;
#16092=ORIENTED_EDGE ( 'NONE', *, *, #12699, .T. ) ;
#16098=ORIENTED_EDGE ( 'NONE', *, *, #28577, .T. ) ;
#16109=EDGE_CURVE ( 'NONE', #4123, #33439, #384, .T. ) ;
#16120=LINE ( 'NONE', #6099, #18439 ) ;
#16121=CARTESIAN_POINT ( 'NONE',  ( -91.72768752788732627, -10.75000000000000000, -57.39251435732919049 ) ) ;
#16147=ORIENTED_EDGE ( 'NONE', *, *, #29057, .T. ) ;
#16154=EDGE_CURVE ( 'NONE', #35877, #22296, #4926, .T. ) ;
#16197=ORIENTED_EDGE ( 'NONE', *, *, #36859, .F. ) ;
#16198=CARTESIAN_POINT ( 'NONE',  ( 22.99999999999999645, 1.749999999999999778, -45.99999999999998579 ) ) ;
#16319=FACE_OUTER_BOUND ( 'NONE', #10109, .T. ) ;
#16339=CARTESIAN_POINT ( 'NONE',  ( -17.89728711128011795, -4.500000000000000000, 51.00000000000000711 ) ) ;
#16388=ORIENTED_EDGE ( 'NONE', *, *, #17119, .T. ) ;
#16389=CARTESIAN_POINT ( 'NONE',  ( -2.668805347656625298E-15, -4.500000000000000000, 40.00000000000002132 ) ) ;
#16449=CARTESIAN_POINT ( 'NONE',  ( 22.99999999999999645, -3.250000000000000444, -45.99999999999998579 ) ) ;
#16484=VECTOR ( 'NONE', #6341, 1000.000000000000000 ) ;
#16507=ORIENTED_EDGE ( 'NONE', *, *, #36702, .T. ) ;
#16527=DIRECTION ( 'NONE',  ( -1.000000000000000000, 0.000000000000000000, 2.242192981248496244E-16 ) ) ;
#16551=CARTESIAN_POINT ( 'NONE',  ( -91.72768752788732627, -10.75000000000000000, -57.39251435732919049 ) ) ;
#16560=VERTEX_POINT ( 'NONE', #2784 ) ;
#16578=CARTESIAN_POINT ( 'NONE',  ( 16.52764414336284915, -15.28760839975256758, 37.82908593122558472 ) ) ;
#16588=DIRECTION ( 'NONE',  ( 0.000000000000000000, -0.000000000000000000, -1.000000000000000000 ) ) ;
#16599=DIRECTION ( 'NONE',  ( 0.000000000000000000, 0.000000000000000000, -1.000000000000000000 ) ) ;
#16623=DIRECTION ( 'NONE',  ( 0.000000000000000000, 0.000000000000000000, 1.000000000000000000 ) ) ;
#16626=VECTOR ( 'NONE', #27454, 1000.000000000000000 ) ;
#16681=PLANE ( 'NONE',  #21902 ) ;
#16701=ORIENTED_EDGE ( 'NONE', *, *, #24448, .F. ) ;
#16769=ORIENTED_EDGE ( 'NONE', *, *, #7141, .T. ) ;
#16771=FACE_BOUND ( 'NONE', #32336, .T. ) ;
#16801=PLANE ( 'NONE',  #27477 ) ;
#16818=EDGE_CURVE ( 'NONE', #33439, #34910, #17403, .T. ) ;
#16821=EDGE_CURVE ( 'NONE', #14257, #32851, #38723, .T. ) ;
#16827=DIRECTION ( 'NONE',  ( 0.000000000000000000, -1.000000000000000000, 0.000000000000000000 ) ) ;
#16847=DIRECTION ( 'NONE',  ( 0.000000000000000000, -1.000000000000000000, 0.000000000000000000 ) ) ;
#16849=DIRECTION ( 'NONE',  ( 0.9643627188534427130, 0.000000000000000000, -0.2645837230171119159 ) ) ;
#16866=DIRECTION ( 'NONE',  ( -0.000000000000000000, 1.000000000000000000, -0.000000000000000000 ) ) ;
#16873=( NAMED_UNIT ( * ) SI_UNIT ( $, .STERADIAN. ) SOLID_ANGLE_UNIT ( ) );
#16885=CARTESIAN_POINT ( 'NONE',  ( 4.257384923554910827, -14.66919072256743561, 44.19375250200204164 ) ) ;
#16898=EDGE_CURVE ( 'NONE', #33170, #13500, #30782, .T. ) ;
#16992=CARTESIAN_POINT ( 'NONE',  ( 16.10157638013081183, -15.38763959456531438, 38.40479877781251616 ) ) ;
#17029=ORIENTED_EDGE ( 'NONE', *, *, #17069, .T. ) ;
#17058=CARTESIAN_POINT ( 'NONE',  ( -1.027389493830889214E-15, 1.750000000000001554, 32.19375250200202743 ) ) ;
#17060=DIRECTION ( 'NONE',  ( -1.000000000000000000, -0.000000000000000000, -2.102695122396128930E-16 ) ) ;
#17069=EDGE_CURVE ( 'NONE', #21499, #2398, #35018, .T. ) ;
#17108=AXIS2_PLACEMENT_3D ( 'NONE', #2916, #22898, #15905 ) ;
#17119=EDGE_CURVE ( 'NONE', #41416, #33277, #33988, .T. ) ;
#17126=EDGE_LOOP ( 'NONE', ( #1341, #14824, #3717, #40403 ) ) ;
#17136=AXIS2_PLACEMENT_3D ( 'NONE', #41599, #35829, #18630 ) ;
#17148=CIRCLE ( 'NONE', #36861, 10.00000000000000178 ) ;
#17149=DIRECTION ( 'NONE',  ( -2.768405754343413644E-16, 0.000000000000000000, -1.000000000000000000 ) ) ;
#17158=CIRCLE ( 'NONE', #7659, 108.2919410404669378 ) ;
#17165=ORIENTED_EDGE ( 'NONE', *, *, #34631, .F. ) ;
#17180=ORIENTED_EDGE ( 'NONE', *, *, #22005, .T. ) ;
#17192=ORIENTED_EDGE ( 'NONE', *, *, #20130, .F. ) ;
#17202=LINE ( 'NONE', #1041, #38652 ) ;
#17207=CARTESIAN_POINT ( 'NONE',  ( 4.257384923554910827, -14.66919072256743561, 44.19375250200204164 ) ) ;
#17221=LINE ( 'NONE', #30185, #9479 ) ;
#17228=VECTOR ( 'NONE', #14866, 1000.000000000000000 ) ;
#17237=EDGE_LOOP ( 'NONE', ( #8940, #2361, #15090, #5336 ) ) ;
#17277=VECTOR ( 'NONE', #27472, 1000.000000000000114 ) ;
#17290=ORIENTED_EDGE ( 'NONE', *, *, #18907, .F. ) ;
#17298=EDGE_CURVE ( 'NONE', #26548, #15664, #12893, .T. ) ;
#17310=FACE_OUTER_BOUND ( 'NONE', #5039, .T. ) ;
#17332=AXIS2_PLACEMENT_3D ( 'NONE', #18765, #22576, #29149 ) ;
#17377=ORIENTED_EDGE ( 'NONE', *, *, #21800, .F. ) ;
#17403=LINE ( 'NONE', #1236, #12242 ) ;
#17446=CARTESIAN_POINT ( 'NONE',  ( 16.03425889574251428, -3.250000000000000444, -46.69170143013996466 ) ) ;
#17483=DIRECTION ( 'NONE',  ( 0.000000000000000000, 1.000000000000000000, 0.000000000000000000 ) ) ;
#17500=VERTEX_POINT ( 'NONE', #4146 ) ;
#17529=ORIENTED_EDGE ( 'NONE', *, *, #11575, .T. ) ;
#17531=CARTESIAN_POINT ( 'NONE',  ( 4.257384923554909051, 7.250000000000000000, 29.19375250200204164 ) ) ;
#17550=DIRECTION ( 'NONE',  ( -0.9643627188534427130, 0.000000000000000000, 0.2645837230171119159 ) ) ;
#17634=ADVANCED_FACE ( 'NONE', ( #29884 ), #11371, .F. ) ;
#17635=VERTEX_POINT ( 'NONE', #30730 ) ;
#17642=CARTESIAN_POINT ( 'NONE',  ( -9.651066704802783391, -14.21913021669518074, 34.82870031257356658 ) ) ;
#17693=AXIS2_PLACEMENT_3D ( 'NONE', #6766, #19740, #25716 ) ;
#17694=DIRECTION ( 'NONE',  ( 0.000000000000000000, -1.000000000000000000, 0.000000000000000000 ) ) ;
#17699=ORIENTED_EDGE ( 'NONE', *, *, #26393, .T. ) ;
#17753=ORIENTED_EDGE ( 'NONE', *, *, #17298, .F. ) ;
#17755=ORIENTED_EDGE ( 'NONE', *, *, #20130, .T. ) ;
#17759=DIRECTION ( 'NONE',  ( -0.2645837230171119159, 0.000000000000000000, -0.9643627188534427130 ) ) ;
#17799=ORIENTED_EDGE ( 'NONE', *, *, #30284, .F. ) ;
#17826=DIRECTION ( 'NONE',  ( 0.000000000000000000, -1.000000000000000000, 0.000000000000000000 ) ) ;
#17843=DIRECTION ( 'NONE',  ( 0.000000000000000000, -1.000000000000000000, 0.000000000000000000 ) ) ;
#17895=DIRECTION ( 'NONE',  ( -1.000000000000000000, -0.000000000000000000, -2.102695122396128930E-16 ) ) ;
#17915=AXIS2_PLACEMENT_3D ( 'NONE', #40432, #34051, #11291 ) ;
#18016=CARTESIAN_POINT ( 'NONE',  ( 4.257384923554909051, 0.8500000000000009770, 29.19375250200204164 ) ) ;
#18026=ORIENTED_EDGE ( 'NONE', *, *, #3833, .T. ) ;
#18053=CARTESIAN_POINT ( 'NONE',  ( -10.00686509496360088, -13.61544027540983670, 33.83855767824705651 ) ) ;
#18070=ADVANCED_FACE ( 'NONE', ( #30677 ), #1128, .F. ) ;
#18074=ORIENTED_EDGE ( 'NONE', *, *, #11993, .F. ) ;
#18130=VERTEX_POINT ( 'NONE', #761 ) ;
#18190=DIRECTION ( 'NONE',  ( -0.9643627188534427130, 0.000000000000000000, 0.2645837230171119159 ) ) ;
#18238=LINE ( 'NONE', #2285, #34076 ) ;
#18243=DIRECTION ( 'NONE',  ( 0.9643627188534427130, 0.000000000000000000, -0.2645837230171117493 ) ) ;
#18334=VECTOR ( 'NONE', #39377, 1000.000000000000000 ) ;
#18366=DIRECTION ( 'NONE',  ( 0.000000000000000000, 0.000000000000000000, 1.000000000000000000 ) ) ;
#18375=ORIENTED_EDGE ( 'NONE', *, *, #21800, .T. ) ;
#18388=CARTESIAN_POINT ( 'NONE',  ( 14.23381301606215743, -5.749999999999999112, -13.75869656311284217 ) ) ;
#18400=LINE ( 'NONE', #14797, #40204 ) ;
#18423=ORIENTED_EDGE ( 'NONE', *, *, #1501, .T. ) ;
#18425=EDGE_LOOP ( 'NONE', ( #20465, #11009, #7927, #11415 ) ) ;
#18430=AXIS2_PLACEMENT_3D ( 'NONE', #38092, #8948, #22138 ) ;
#18439=VECTOR ( 'NONE', #6314, 1000.000000000000000 ) ;
#18534=VERTEX_POINT ( 'NONE', #41786 ) ;
#18555=DIRECTION ( 'NONE',  ( 0.000000000000000000, 0.000000000000000000, 1.000000000000000000 ) ) ;
#18601=VECTOR ( 'NONE', #14715, 1000.000000000000000 ) ;
#18609=CARTESIAN_POINT ( 'NONE',  ( 13.19971406886381615, -9.749999999999998224, -9.306493635776055484 ) ) ;
#18611=CARTESIAN_POINT ( 'NONE',  ( -2.668805347656625298E-15, -4.500000000000000000, 40.00000000000002132 ) ) ;
#18630=DIRECTION ( 'NONE',  ( 0.000000000000000000, 0.000000000000000000, -1.000000000000000000 ) ) ;
#18636=AXIS2_PLACEMENT_3D ( 'NONE', #16389, #26170, #12553 ) ;
#18670=CARTESIAN_POINT ( 'NONE',  ( 33.00000000000001421, -4.500000000000000000, 44.00000000000003553 ) ) ;
#18713=DIRECTION ( 'NONE',  ( -0.2262442655067633257, 0.000000000000000000, 0.9740705992510528821 ) ) ;
#18740=CARTESIAN_POINT ( 'NONE',  ( 18.17327386434068970, 4.087762173755774775, 34.83183720942130179 ) ) ;
#18741=ORIENTED_EDGE ( 'NONE', *, *, #32104, .T. ) ;
#18765=CARTESIAN_POINT ( 'NONE',  ( 22.99999999999999645, -10.75000000000000000, -45.99999999999998579 ) ) ;
#18797=EDGE_LOOP ( 'NONE', ( #28089, #23130, #14511, #7338, #41189, #32538 ) ) ;
#18874=FACE_OUTER_BOUND ( 'NONE', #1064, .T. ) ;
#18886=LINE ( 'NONE', #15706, #2173 ) ;
#18898=ORIENTED_EDGE ( 'NONE', *, *, #14150, .F. ) ;
#18907=EDGE_CURVE ( 'NONE', #38940, #7337, #38165, .T. ) ;
#18914=DIRECTION ( 'NONE',  ( -0.9740705992510528821, 0.000000000000000000, -0.2262442655067633257 ) ) ;
#18944=ORIENTED_EDGE ( 'NONE', *, *, #1190, .F. ) ;
#18954=PLANE ( 'NONE',  #26718 ) ;
#18976=DIRECTION ( 'NONE',  ( -0.000000000000000000, 1.000000000000000000, -0.000000000000000000 ) ) ;
#18994=DIRECTION ( 'NONE',  ( 0.000000000000000000, 0.000000000000000000, 1.000000000000000000 ) ) ;
#18998=CARTESIAN_POINT ( 'NONE',  ( -33.00000000000001421, 1.750000000000001554, 32.19375250200204164 ) ) ;
#19014=PLANE ( 'NONE',  #31191 ) ;
#19066=CARTESIAN_POINT ( 'NONE',  ( 4.257384923554909939, 7.250000000000000000, 23.69375250200204874 ) ) ;
#19079=DIRECTION ( 'NONE',  ( -0.08163352362547933450, 0.000000000000000000, -0.9966624141706600382 ) ) ;
#19081=FACE_OUTER_BOUND ( 'NONE', #3713, .T. ) ;
#19112=ORIENTED_EDGE ( 'NONE', *, *, #38170, .T. ) ;
#19117=DIRECTION ( 'NONE',  ( -1.000000000000000000, -0.000000000000000000, -2.102695122396128930E-16 ) ) ;
#19156=CARTESIAN_POINT ( 'NONE',  ( 4.257384923554909051, 7.250000000000000000, 29.19375250200204164 ) ) ;
#19162=ORIENTED_EDGE ( 'NONE', *, *, #534, .T. ) ;
#19165=CARTESIAN_POINT ( 'NONE',  ( 22.99999999999999645, -3.250000000000000444, -45.99999999999998579 ) ) ;
#19168=ORIENTED_EDGE ( 'NONE', *, *, #13164, .F. ) ;
#19169=DIRECTION ( 'NONE',  ( 0.000000000000000000, 0.000000000000000000, -1.000000000000000000 ) ) ;
#19215=CIRCLE ( 'NONE', #24629, 10.00000000000000178 ) ;
#19240=CARTESIAN_POINT ( 'NONE',  ( 22.99999999999999645, -5.749999999999999112, -52.99999999999997868 ) ) ;
#19271=EDGE_CURVE ( 'NONE', #8412, #16560, #12849, .T. ) ;
#19323=CARTESIAN_POINT ( 'NONE',  ( 17.89728711128010374, -4.500000000000000000, 51.00000000000000711 ) ) ;
#19341=CARTESIAN_POINT ( 'NONE',  ( -0.5118368542555185030, 5.952454039762226756, 43.44862648885644063 ) ) ;
#19357=EDGE_LOOP ( 'NONE', ( #17377, #7446, #10096, #34584 ) ) ;
#19362=EDGE_LOOP ( 'NONE', ( #39869, #8287 ) ) ;
#19371=EDGE_LOOP ( 'NONE', ( #28409, #32480, #9122, #7110, #35098 ) ) ;
#19372=FACE_OUTER_BOUND ( 'NONE', #23397, .T. ) ;
#19387=DIRECTION ( 'NONE',  ( 0.000000000000000000, -1.000000000000000000, 0.000000000000000000 ) ) ;
#19393=LINE ( 'NONE', #6000, #13260 ) ;
#19408=DIRECTION ( 'NONE',  ( 0.000000000000000000, -0.000000000000000000, -1.000000000000000000 ) ) ;
#19496=CARTESIAN_POINT ( 'NONE',  ( -33.00000000000002132, -4.499999999999999112, 35.99999999999998579 ) ) ;
#19505=CARTESIAN_POINT ( 'NONE',  ( 14.23381301606215565, -9.749999999999998224, -13.75869656311283151 ) ) ;
#19516=EDGE_CURVE ( 'NONE', #7535, #3004, #21142, .T. ) ;
#19546=CARTESIAN_POINT ( 'NONE',  ( -10.57407137268529596, 2.556825748764473438, 31.50514758954957983 ) ) ;
#19564=CARTESIAN_POINT ( 'NONE',  ( 16.03425889574251428, -5.749999999999999112, -46.69170143013996466 ) ) ;
#19602=CIRCLE ( 'NONE', #8740, 105.2919410404669520 ) ;
#19606=CARTESIAN_POINT ( 'NONE',  ( -33.00000000000002842, -4.500000000000000000, 40.00000000000001421 ) ) ;
#19619=ORIENTED_EDGE ( 'NONE', *, *, #8994, .F. ) ;
#19630=AXIS2_PLACEMENT_3D ( 'NONE', #8470, #17843, #11450 ) ;
#19638=EDGE_CURVE ( 'NONE', #30663, #569, #6199, .T. ) ;
#19727=DIRECTION ( 'NONE',  ( -0.000000000000000000, 1.000000000000000000, -0.000000000000000000 ) ) ;
#19740=DIRECTION ( 'NONE',  ( -3.672050975999536074E-16, 0.000000000000000000, -1.000000000000000000 ) ) ;
#19753=CARTESIAN_POINT ( 'NONE',  ( 14.66652723975663442, -15.51022990707443938, 40.01826027516346329 ) ) ;
#19770=VERTEX_POINT ( 'NONE', #4487 ) ;
#19792=AXIS2_PLACEMENT_3D ( 'NONE', #24219, #14016, #29952 ) ;
#19804=CYLINDRICAL_SURFACE ( 'NONE', #26651, 5.499999999999991118 ) ;
#19830=ADVANCED_FACE ( 'NONE', ( #37033 ), #27038, .T. ) ;
#19857=CARTESIAN_POINT ( 'NONE',  ( 17.89728711128010374, -4.500000000000000000, 50.00000000000001421 ) ) ;
#19881=ORIENTED_EDGE ( 'NONE', *, *, #20992, .F. ) ;
#19890=CARTESIAN_POINT ( 'NONE',  ( -26.68952268848979870, -5.749999999999999112, 29.19375250200205230 ) ) ;
#19928=ORIENTED_EDGE ( 'NONE', *, *, #31455, .T. ) ;
#19956=DIRECTION ( 'NONE',  ( -1.000000000000000000, -0.000000000000000000, -2.102695122396128930E-16 ) ) ;
#20008=ORIENTED_EDGE ( 'NONE', *, *, #4821, .F. ) ;
#20037=VECTOR ( 'NONE', #31356, 999.9999999999998863 ) ;
#20056=CARTESIAN_POINT ( 'NONE',  ( 29.99999999999999645, -3.250000000000000444, -45.99999999999998579 ) ) ;
#20095=AXIS2_PLACEMENT_3D ( 'NONE', #28775, #22400, #15831 ) ;
#20130=EDGE_CURVE ( 'NONE', #29227, #35877, #4645, .T. ) ;
#20144=EDGE_CURVE ( 'NONE', #39224, #34910, #33580, .T. ) ;
#20153=LINE ( 'NONE', #3555, #13044 ) ;
#20182=EDGE_CURVE ( 'NONE', #35010, #18130, #1249, .T. ) ;
#20183=CARTESIAN_POINT ( 'NONE',  ( 16.72779263771517222, -15.22507417841562294, 37.53709948269236918 ) ) ;
#20187=CARTESIAN_POINT ( 'NONE',  ( 29.99999999999999645, 1.749999999999999778, -45.99999999999998579 ) ) ;
#20196=DIRECTION ( 'NONE',  ( 0.000000000000000000, -1.000000000000000000, 0.000000000000000000 ) ) ;
#20213=ADVANCED_FACE ( 'NONE', ( #30799 ), #11237, .F. ) ;
#20216=EDGE_LOOP ( 'NONE', ( #2371, #10317, #11722, #12413, #20978, #9924, #34180, #41396, #28302, #15975, #5589, #41558, #19881, #8423, #33899, #28885, #10737 ) ) ;
#20249=CARTESIAN_POINT ( 'NONE',  ( 4.257384923554909051, -9.749999999999998224, 14.19375250200204341 ) ) ;
#20274=EDGE_CURVE ( 'NONE', #7337, #39599, #25049, .T. ) ;
#20296=CARTESIAN_POINT ( 'NONE',  ( 4.257384923554909051, 0.8500000000000009770, 29.19375250200204164 ) ) ;
#20349=ORIENTED_EDGE ( 'NONE', *, *, #24056, .F. ) ;
#20392=CARTESIAN_POINT ( 'NONE',  ( 4.976097163484448416, -14.66919072256743384, 44.19375250200203453 ) ) ;
#20421=ORIENTED_EDGE ( 'NONE', *, *, #37884, .T. ) ;
#20427=EDGE_CURVE ( 'NONE', #24045, #37673, #18238, .T. ) ;
#20457=PLANE ( 'NONE',  #40806 ) ;
#20464=DIRECTION ( 'NONE',  ( -0.000000000000000000, -1.000000000000000000, -0.000000000000000000 ) ) ;
#20465=ORIENTED_EDGE ( 'NONE', *, *, #24096, .F. ) ;
#20473=AXIS2_PLACEMENT_3D ( 'NONE', #19156, #32126, #21713 ) ;
#20511=EDGE_CURVE ( 'NONE', #34649, #37673, #16120, .T. ) ;
#20522=VECTOR ( 'NONE', #13187, 1000.000000000000000 ) ;
#20533=DIRECTION ( 'NONE',  ( 0.000000000000000000, 0.000000000000000000, 1.000000000000000000 ) ) ;
#20543=FACE_OUTER_BOUND ( 'NONE', #4419, .T. ) ;
#20575=ORIENTED_EDGE ( 'NONE', *, *, #24708, .T. ) ;
#20583=ORIENTED_EDGE ( 'NONE', *, *, #12137, .T. ) ;
#20595=DIRECTION ( 'NONE',  ( 0.000000000000000000, 0.000000000000000000, 1.000000000000000000 ) ) ;
#20619=VECTOR ( 'NONE', #18190, 1000.000000000000114 ) ;
#20629=CIRCLE ( 'NONE', #26764, 4.000000000000031086 ) ;
#20640=VECTOR ( 'NONE', #16847, 1000.000000000000000 ) ;
#20676=EDGE_CURVE ( 'NONE', #35010, #32751, #35440, .T. ) ;
#20752=DIRECTION ( 'NONE',  ( 2.768405754343413644E-16, 0.000000000000000000, 1.000000000000000000 ) ) ;
#20783=AXIS2_PLACEMENT_3D ( 'NONE', #12200, #38152, #11778 ) ;
#20834=CARTESIAN_POINT ( 'NONE',  ( -3.160957784022181194, -15.27745473971046053, 42.26750874438840810 ) ) ;
#20838=FACE_BOUND ( 'NONE', #11986, .T. ) ;
#20843=ORIENTED_EDGE ( 'NONE', *, *, #19516, .T. ) ;
#20860=LINE ( 'NONE', #1297, #26139 ) ;
#20904=CARTESIAN_POINT ( 'NONE',  ( 13.19971406886381793, -3.250000000000000444, -9.306493635776062590 ) ) ;
#20964=CARTESIAN_POINT ( 'NONE',  ( 22.99999999999999645, -9.749999999999998224, -52.99999999999997868 ) ) ;
#20978=ORIENTED_EDGE ( 'NONE', *, *, #3548, .F. ) ;
#20981=CARTESIAN_POINT ( 'NONE',  ( -26.68952268848979870, -3.250000000000000444, 29.19375250200205230 ) ) ;
#20992=EDGE_CURVE ( 'NONE', #24287, #33538, #18400, .T. ) ;
#20997=ORIENTED_EDGE ( 'NONE', *, *, #22562, .T. ) ;
#21017=DIRECTION ( 'NONE',  ( -0.2262442655067632979, 0.000000000000000000, 0.9740705992510528821 ) ) ;
#21035=CARTESIAN_POINT ( 'NONE',  ( -9.286862925412830094, -14.60322692305086356, 35.64404424871759147 ) ) ;
#21046=AXIS2_PLACEMENT_3D ( 'NONE', #34827, #5694, #18243 ) ;
#21096=CARTESIAN_POINT ( 'NONE',  ( -11.21606888246744127, -3.250000000000000444, 29.19375250200204519 ) ) ;
#21142=CIRCLE ( 'NONE', #2801, 5.499999999999991118 ) ;
#21148=ORIENTED_EDGE ( 'NONE', *, *, #7232, .T. ) ;
#21186=CARTESIAN_POINT ( 'NONE',  ( -91.72768752788732627, -5.749999999999999112, -57.39251435732919049 ) ) ;
#21211=CARTESIAN_POINT ( 'NONE',  ( 7.651048906156359131, -3.250000000000000444, 14.58269351323623830 ) ) ;
#21238=PLANE ( 'NONE',  #35517 ) ;
#21241=CARTESIAN_POINT ( 'NONE',  ( -8.383326646241526348, -15.16687753108797665, 37.28331021637578857 ) ) ;
#21244=ADVANCED_FACE ( 'NONE', ( #40749 ), #11816, .T. ) ;
#21253=CIRCLE ( 'NONE', #41628, 15.00000000000000000 ) ;
#21343=VERTEX_POINT ( 'NONE', #8629 ) ;
#21348=LINE ( 'NONE', #2411, #40887 ) ;
#21459=ORIENTED_EDGE ( 'NONE', *, *, #39172, .T. ) ;
#21470=EDGE_CURVE ( 'NONE', #30209, #39425, #32015, .T. ) ;
#21499=VERTEX_POINT ( 'NONE', #98 ) ;
#21518=CARTESIAN_POINT ( 'NONE',  ( 22.99999999999999645, -10.75000000000000000, -45.99999999999998579 ) ) ;
#21523=ADVANCED_FACE ( 'NONE', ( #29027 ), #9905, .T. ) ;
#21530=ADVANCED_FACE ( 'NONE', ( #38818 ), #22861, .T. ) ;
#21554=DIRECTION ( 'NONE',  ( 1.000000000000000000, 0.000000000000000000, 2.102695122396128930E-16 ) ) ;
#21586=FACE_OUTER_BOUND ( 'NONE', #35436, .T. ) ;
#21602=CARTESIAN_POINT ( 'NONE',  ( 16.03425889574251428, -10.75000000000000000, -46.69170143013996466 ) ) ;
#21603=DIRECTION ( 'NONE',  ( 0.000000000000000000, -0.000000000000000000, -1.000000000000000000 ) ) ;
#21618=EDGE_CURVE ( 'NONE', #22195, #39425, #4313, .T. ) ;
#21638=FACE_OUTER_BOUND ( 'NONE', #3914, .T. ) ;
#21639=LINE ( 'NONE', #5696, #32963 ) ;
#21648=DIRECTION ( 'NONE',  ( 0.000000000000000000, -1.000000000000000000, 0.000000000000000000 ) ) ;
#21660=EDGE_CURVE ( 'NONE', #12249, #11862, #22558, .T. ) ;
#21695=FACE_OUTER_BOUND ( 'NONE', #35544, .T. ) ;
#21701=VECTOR ( 'NONE', #7652, 1000.000000000000000 ) ;
#21705=VERTEX_POINT ( 'NONE', #20056 ) ;
#21711=B_SPLINE_CURVE_WITH_KNOTS ( 'NONE', 3,
 ( #11655, #5282, #31227, #27625, #24442, #1679, #24033, #15072, #20834, #4661, #8061, #5073, #37409, #14449, #8267, #21241, #11254, #27425, #37206, #21035, #24237, #17642, #34213, #18053, #31027, #37614, #2721, #22491, #15924, #12509 ),
 .UNSPECIFIED., .F., .F.,
 ( 4, 2, 2, 2, 2, 2, 2, 2, 2, 2, 2, 2, 2, 2, 4 ),
 ( 0.01718506176362324944, 0.02009064427908128017, 0.02154343553681029727, 0.02299622679453931090, 0.02590180930999734857, 0.02880739182545538624, 0.03026018308318440334, 0.03171297434091342043, 0.03316576559864244100, 0.03389216122750693394, 0.03461855685637144076, 0.03607134811410045439, 0.03679774374296494732, 0.03752413937182944720, 0.04042972188728742589 ),
 .UNSPECIFIED. ) ;
#21713=DIRECTION ( 'NONE',  ( 0.000000000000000000, 0.000000000000000000, 1.000000000000000000 ) ) ;
#21721=ORIENTED_EDGE ( 'NONE', *, *, #8037, .T. ) ;
#21743=VECTOR ( 'NONE', #28001, 1000.000000000000000 ) ;
#21753=LINE ( 'NONE', #5594, #5143 ) ;
#21777=PRODUCT ( 'Aluminum Fixing Part', 'Aluminum Fixing Part', '', ( #522 ) ) ;
#21800=EDGE_CURVE ( 'NONE', #17635, #11308, #15142, .T. ) ;
#21815=FACE_OUTER_BOUND ( 'NONE', #23403, .T. ) ;
#21829=CYLINDRICAL_SURFACE ( 'NONE', #15828, 9.999999999999980460 ) ;
#21837=VECTOR ( 'NONE', #23590, 1000.000000000000000 ) ;
#21846=CARTESIAN_POINT ( 'NONE',  ( -26.68952268848979870, -10.75000000000000000, 29.19375250200205230 ) ) ;
#21877=AXIS2_PLACEMENT_3D ( 'NONE', #40358, #37173, #8026 ) ;
#21902=AXIS2_PLACEMENT_3D ( 'NONE', #19857, #29851, #26459 ) ;
#21910=LINE ( 'NONE', #11919, #15920 ) ;
#21928=DIRECTION ( 'NONE',  ( -0.000000000000000000, 1.000000000000000000, -0.000000000000000000 ) ) ;
#21934=CARTESIAN_POINT ( 'NONE',  ( 30.00000000000000000, -5.749999999999998224, -18.08432671081678578 ) ) ;
#21969=CARTESIAN_POINT ( 'NONE',  ( 32.99999999999999289, 1.750000000000001554, -45.99999999999999289 ) ) ;
#22005=EDGE_CURVE ( 'NONE', #30209, #29227, #33130, .T. ) ;
#22045=ADVANCED_FACE ( 'NONE', ( #16771, #38520 ), #3995, .F. ) ;
#22057=UNCERTAINTY_MEASURE_WITH_UNIT (LENGTH_MEASURE( 1.000000000000000082E-05 ), #119, 'distance_accuracy_value', 'NONE');
#22060=AXIS2_PLACEMENT_3D ( 'NONE', #37851, #18914, #18713 ) ;
#22068=LINE ( 'NONE', #12493, #14251 ) ;
#22071=DIRECTION ( 'NONE',  ( 0.000000000000000000, 1.000000000000000000, 0.000000000000000000 ) ) ;
#22075=VECTOR ( 'NONE', #4431, 1000.000000000000000 ) ;
#22099=CARTESIAN_POINT ( 'NONE',  ( 17.09591398984245458, 6.075650775949320348, 36.95876640613690256 ) ) ;
#22138=DIRECTION ( 'NONE',  ( 1.000000000000000000, 0.000000000000000000, -3.672050975999536074E-16 ) ) ;
#22195=VERTEX_POINT ( 'NONE', #21211 ) ;
#22250=ORIENTED_EDGE ( 'NONE', *, *, #16898, .F. ) ;
#22296=VERTEX_POINT ( 'NONE', #33344 ) ;
#22301=DIRECTION ( 'NONE',  ( -3.469446951953618626E-16, 0.000000000000000000, 1.000000000000000000 ) ) ;
#22306=CIRCLE ( 'NONE', #13570, 108.2919410404669378 ) ;
#22335=EDGE_CURVE ( 'NONE', #3004, #12249, #12476, .T. ) ;
#22378=FACE_OUTER_BOUND ( 'NONE', #3100, .T. ) ;
#22384=STYLED_ITEM('',(#42145),#22626);
#22389=EDGE_CURVE ( 'NONE', #5666, #18534, #15259, .T. ) ;
#22397=ORIENTED_EDGE ( 'NONE', *, *, #11613, .F. ) ;
#22400=DIRECTION ( 'NONE',  ( -0.000000000000000000, 1.000000000000000000, -0.000000000000000000 ) ) ;
#22408=VECTOR ( 'NONE', #11303, 1000.000000000000000 ) ;
#22446=ORIENTED_EDGE ( 'NONE', *, *, #17069, .F. ) ;
#22452=CARTESIAN_POINT ( 'NONE',  ( 4.257384923554909051, 0.8500000000000009770, 39.93125250200203880 ) ) ;
#22456=DIRECTION ( 'NONE',  ( -1.000000000000000000, -0.000000000000000000, -2.102695122396128930E-16 ) ) ;
#22478=CARTESIAN_POINT ( 'NONE',  ( 7.651048906156357354, -9.749999999999998224, 14.58269351323625074 ) ) ;
#22489=CARTESIAN_POINT ( 'NONE',  ( 22.99999999999999645, -9.749999999999998224, -45.99999999999998579 ) ) ;
#22491=CARTESIAN_POINT ( 'NONE',  ( -10.46653695873021128, -12.27157421205372323, 32.15630662161991182 ) ) ;
#22510=CARTESIAN_POINT ( 'NONE',  ( 8.155924269577814911, 5.865759273864133760, 43.68274915641599421 ) ) ;
#22524=CARTESIAN_POINT ( 'NONE',  ( -10.00832803044954211, 4.612372513095444049, 33.83403948934240901 ) ) ;
#22547=VECTOR ( 'NONE', #1821, 1000.000000000000000 ) ;
#22556=ORIENTED_EDGE ( 'NONE', *, *, #20182, .F. ) ;
#22558=CIRCLE ( 'NONE', #4234, 5.499999999999991118 ) ;
#22562=EDGE_CURVE ( 'NONE', #30721, #39665, #9714, .T. ) ;
#22576=DIRECTION ( 'NONE',  ( 0.000000000000000000, -1.000000000000000000, 0.000000000000000000 ) ) ;
#22598=LINE ( 'NONE', #23012, #18334 ) ;
#22626=MANIFOLD_SOLID_BREP ( 'Boss-Extrude12', #39630 ) ;
#22654=DIRECTION ( 'NONE',  ( -1.000000000000000000, -0.000000000000000000, -2.102695122396128930E-16 ) ) ;
#22668=CARTESIAN_POINT ( 'NONE',  ( -91.72768752788732627, -9.749999999999998224, -57.39251435732919049 ) ) ;
#22715=PLANE ( 'NONE',  #1998 ) ;
#22739=CARTESIAN_POINT ( 'NONE',  ( 13.56948360559098710, -15.46031462669751555, 40.95874692614047063 ) ) ;
#22740=EDGE_CURVE ( 'NONE', #21705, #22296, #14365, .T. ) ;
#22757=ORIENTED_EDGE ( 'NONE', *, *, #22335, .T. ) ;
#22758=CYLINDRICAL_SURFACE ( 'NONE', #18636, 4.000000000000017764 ) ;
#22861=CYLINDRICAL_SURFACE ( 'NONE', #17136, 10.00000000000000178 ) ;
#22898=DIRECTION ( 'NONE',  ( -1.000000000000000000, -0.000000000000000000, -2.102695122396128930E-16 ) ) ;
#22935=PLANE ( 'NONE',  #17693 ) ;
#22945=DIRECTION ( 'NONE',  ( 0.000000000000000000, 0.000000000000000000, 1.000000000000000000 ) ) ;
#22949=CARTESIAN_POINT ( 'NONE',  ( -7.848366639703233893, 6.335808145850082340, 38.06391143773804231 ) ) ;
#22955=PLANE ( 'NONE',  #5002 ) ;
#22965=DIRECTION ( 'NONE',  ( 0.000000000000000000, 1.000000000000000000, 0.000000000000000000 ) ) ;
#22974=ADVANCED_FACE ( 'NONE', ( #2636 ), #19014, .F. ) ;
#23012=CARTESIAN_POINT ( 'NONE',  ( -26.68952268848979870, 1.749999999999999778, 29.19375250200205230 ) ) ;
#23080=DIRECTION ( 'NONE',  ( -1.000000000000000000, -0.000000000000000000, -2.102695122396128930E-16 ) ) ;
#23117=VECTOR ( 'NONE', #40457, 1000.000000000000000 ) ;
#23130=ORIENTED_EDGE ( 'NONE', *, *, #11806, .T. ) ;
#23154=CARTESIAN_POINT ( 'NONE',  ( 7.820395667581496291, -14.83164961654870773, 43.78187824946888895 ) ) ;
#23159=CIRCLE ( 'NONE', #20473, 10.73749999999999716 ) ;
#23223=CARTESIAN_POINT ( 'NONE',  ( 4.257384923554909051, 0.8500000000000017542, 29.19375250200204164 ) ) ;
#23227=ORIENTED_EDGE ( 'NONE', *, *, #14043, .T. ) ;
#23239=DIRECTION ( 'NONE',  ( -1.000000000000000000, -0.000000000000000000, -2.102695122396128930E-16 ) ) ;
#23275=CARTESIAN_POINT ( 'NONE',  ( 33.00000000000001421, -4.500000000000000000, 40.00000000000002842 ) ) ;
#23286=VERTEX_POINT ( 'NONE', #20904 ) ;
#23315=CARTESIAN_POINT ( 'NONE',  ( -12.28065031820330155, -5.749999999999999112, 16.19629439043522012 ) ) ;
#23346=DIRECTION ( 'NONE',  ( -0.000000000000000000, -1.000000000000000000, -0.000000000000000000 ) ) ;
#23397=EDGE_LOOP ( 'NONE', ( #17290, #16507, #24841, #27112 ) ) ;
#23400=ORIENTED_EDGE ( 'NONE', *, *, #16109, .F. ) ;
#23403=EDGE_LOOP ( 'NONE', ( #22446, #18741, #18026, #23227, #33710, #38019, #8522 ) ) ;
#23405=VECTOR ( 'NONE', #27198, 1000.000000000000000 ) ;
#23445=AXIS2_PLACEMENT_3D ( 'NONE', #16198, #15567, #19169 ) ;
#23447=CARTESIAN_POINT ( 'NONE',  ( 19.25738492355490550, -10.75000000000000000, 29.19375250200203453 ) ) ;
#23540=CARTESIAN_POINT ( 'NONE',  ( 4.257384923554909051, -9.749999999999998224, 29.19375250200204164 ) ) ;
#23546=LINE ( 'NONE', #39904, #34659 ) ;
#23588=CARTESIAN_POINT ( 'NONE',  ( 17.89728711128010374, -4.500000000000000000, 50.00000000000002132 ) ) ;
#23590=DIRECTION ( 'NONE',  ( 0.000000000000000000, 0.000000000000000000, -1.000000000000000000 ) ) ;
#23594=CARTESIAN_POINT ( 'NONE',  ( 9.185037880478883920, -14.97324005117927470, 43.36579448086791899 ) ) ;
#23660=B_SPLINE_CURVE_WITH_KNOTS ( 'NONE', 3,
 ( #36340, #10401, #29955, #20183, #16578, #16992, #828, #13802, #19753, #30170, #22739, #33357, #39747, #29532, #13165, #10614, #3583, #23594, #399, #23154, #36553, #7419, #20392, #17207 ),
 .UNSPECIFIED., .F., .F.,
 ( 4, 2, 2, 2, 2, 2, 2, 2, 2, 2, 2, 4 ),
 ( 0.000000000000000000, 0.002148132720452902277, 0.003222199080679350597, 0.004296265440905799350, 0.006444398161358702928, 0.007518464521585155151, 0.008592530881811607374, 0.01074066360226451182, 0.01181472996249096838, 0.01288879632271742494, 0.01503692904317033806, 0.01718506176362324944 ),
 .UNSPECIFIED. ) ;
#23664=CARTESIAN_POINT ( 'NONE',  ( 11.02911845508759470, -9.749999999999998224, -8.710966395423659137 ) ) ;
#23723=AXIS2_PLACEMENT_3D ( 'NONE', #9216, #41975, #25599 ) ;
#23800=CARTESIAN_POINT ( 'NONE',  ( 23.34627465269464253, -9.749999999999998224, -52.99143003003683816 ) ) ;
#23813=ORIENTED_EDGE ( 'NONE', *, *, #8994, .T. ) ;
#23883=VECTOR ( 'NONE', #14723, 999.9999999999998863 ) ;
#23936=ORIENTED_EDGE ( 'NONE', *, *, #11806, .F. ) ;
#24030=DIRECTION ( 'NONE',  ( 1.178372492411205818E-15, 0.000000000000000000, 1.000000000000000000 ) ) ;
#24032=VECTOR ( 'NONE', #31998, 1000.000000000000000 ) ;
#24033=CARTESIAN_POINT ( 'NONE',  ( -0.9664805169280994424, -15.00661177974181193, 43.26299489605920456 ) ) ;
#24045=VERTEX_POINT ( 'NONE', #23447 ) ;
#24046=VERTEX_POINT ( 'NONE', #20249 ) ;
#24056=EDGE_CURVE ( 'NONE', #29045, #8624, #24088, .T. ) ;
#24082=CARTESIAN_POINT ( 'NONE',  ( -17.89728711128011795, 1.750000000000001554, 30.94806650488419564 ) ) ;
#24088=LINE ( 'NONE', #14086, #14255 ) ;
#24096=EDGE_CURVE ( 'NONE', #34910, #41715, #30661, .T. ) ;
#24104=DIRECTION ( 'NONE',  ( -0.000000000000000000, 1.000000000000000000, -0.000000000000000000 ) ) ;
#24112=DIRECTION ( 'NONE',  ( 0.000000000000000000, 0.000000000000000000, 1.000000000000000000 ) ) ;
#24119=EDGE_CURVE ( 'NONE', #7337, #4123, #10894, .T. ) ;
#24154=CARTESIAN_POINT ( 'NONE',  ( 17.89728711128010730, -13.39722992726008854, 35.43499182679077109 ) ) ;
#24157=ORIENTED_EDGE ( 'NONE', *, *, #30369, .F. ) ;
#24219=CARTESIAN_POINT ( 'NONE',  ( -91.72768752788732627, 1.750000000000001554, -57.39251435732919049 ) ) ;
#24234=LINE ( 'NONE', #27423, #34877 ) ;
#24235=LINE ( 'NONE', #24861, #25082 ) ;
#24237=CARTESIAN_POINT ( 'NONE',  ( -9.382448520356968302, -14.51244950359679287, 35.43909953030242121 ) ) ;
#24287=VERTEX_POINT ( 'NONE', #1931 ) ;
#24310=EDGE_LOOP ( 'NONE', ( #14908, #28680, #14084, #1838 ) ) ;
#24337=LINE ( 'NONE', #33901, #25721 ) ;
#24389=DIRECTION ( 'NONE',  ( 0.000000000000000000, -1.000000000000000000, 0.000000000000000000 ) ) ;
#24404=ADVANCED_FACE ( 'NONE', ( #12767 ), #39326, .T. ) ;
#24405=CARTESIAN_POINT ( 'NONE',  ( -10.74261507644508740, -10.75000000000000000, 29.19375250200204874 ) ) ;
#24411=DIRECTION ( 'NONE',  ( -1.000000000000000000, 0.000000000000000000, -2.102695122396128930E-16 ) ) ;
#24435=CARTESIAN_POINT ( 'NONE',  ( -4.981769982292365592E-15, -4.500000000000000000, 51.00000000000000711 ) ) ;
#24441=CARTESIAN_POINT ( 'NONE',  ( -26.68952268848979870, -5.749999999999999112, 29.19375250200205230 ) ) ;
#24442=CARTESIAN_POINT ( 'NONE',  ( 0.4211840870959887573, -14.85900860563851111, 43.70306366333630876 ) ) ;
#24448=EDGE_CURVE ( 'NONE', #27946, #15662, #7013, .T. ) ;
#24456=CARTESIAN_POINT ( 'NONE',  ( 7.651048906156359131, -5.749999999999999112, 14.58269351323623830 ) ) ;
#24512=DIRECTION ( 'NONE',  ( -1.000000000000000000, -0.000000000000000000, -2.102695122396128930E-16 ) ) ;
#24516=ORIENTED_EDGE ( 'NONE', *, *, #4311, .F. ) ;
#24543=CARTESIAN_POINT ( 'NONE',  ( 4.257384923554909051, -19.75000000000000000, 29.19375250200204164 ) ) ;
#24580=FACE_OUTER_BOUND ( 'NONE', #35102, .T. ) ;
#24601=DIRECTION ( 'NONE',  ( 0.000000000000000000, 0.000000000000000000, -1.000000000000000000 ) ) ;
#24610=VERTEX_POINT ( 'NONE', #3822 ) ;
#24629=AXIS2_PLACEMENT_3D ( 'NONE', #39391, #29184, #38778 ) ;
#24653=CARTESIAN_POINT ( 'NONE',  ( -11.21606888246744482, -5.749999999999999112, 29.19375250200205585 ) ) ;
#24667=DIRECTION ( 'NONE',  ( 0.000000000000000000, 0.000000000000000000, 1.000000000000000000 ) ) ;
#24684=AXIS2_PLACEMENT_3D ( 'NONE', #21518, #21928, #14730 ) ;
#24698=DIRECTION ( 'NONE',  ( 0.000000000000000000, -1.000000000000000000, 0.000000000000000000 ) ) ;
#24707=CARTESIAN_POINT ( 'NONE',  ( 32.99999999999999289, 1.750000000000001554, -45.99999999999999289 ) ) ;
#24708=EDGE_CURVE ( 'NONE', #5713, #36380, #5498, .T. ) ;
#24714=CARTESIAN_POINT ( 'NONE',  ( -11.21606888246744127, 0.7499999999999997780, 29.19375250200204519 ) ) ;
#24729=ORIENTED_EDGE ( 'NONE', *, *, #27143, .F. ) ;
#24783=AXIS2_PLACEMENT_3D ( 'NONE', #15911, #2922, #5481 ) ;
#24793=DIRECTION ( 'NONE',  ( -1.000000000000000000, -0.000000000000000000, -2.102695122396128930E-16 ) ) ;
#24819=VERTEX_POINT ( 'NONE', #11455 ) ;
#24825=EDGE_LOOP ( 'NONE', ( #1839, #20583, #1997, #14507, #30549, #10300 ) ) ;
#24841=ORIENTED_EDGE ( 'NONE', *, *, #1793, .T. ) ;
#24856=ORIENTED_EDGE ( 'NONE', *, *, #12147, .T. ) ;
#24861=CARTESIAN_POINT ( 'NONE',  ( -11.21606888246744127, 0.7499999999999997780, 29.19375250200204519 ) ) ;
#24878=ORIENTED_EDGE ( 'NONE', *, *, #2370, .T. ) ;
#24888=ADVANCED_FACE ( 'NONE', ( #6339 ), #22715, .T. ) ;
#24916=DIRECTION ( 'NONE',  ( -0.000000000000000000, -1.000000000000000000, -0.000000000000000000 ) ) ;
#24939=ORIENTED_EDGE ( 'NONE', *, *, #11575, .F. ) ;
#24959=CARTESIAN_POINT ( 'NONE',  ( 22.99999999999999645, 0.7499999999999997780, -45.99999999999998579 ) ) ;
#24966=EDGE_LOOP ( 'NONE', ( #31446, #1166, #37832, #34701 ) ) ;
#24981=DIRECTION ( 'NONE',  ( -1.000000000000000000, 0.000000000000000000, 3.672050975999536074E-16 ) ) ;
#24989=LINE ( 'NONE', #36978, #20037 ) ;
#24998=DIRECTION ( 'NONE',  ( 0.000000000000000000, -1.000000000000000000, 0.000000000000000000 ) ) ;
#25029=ORIENTED_EDGE ( 'NONE', *, *, #40650, .T. ) ;
#25035=DIRECTION ( 'NONE',  ( 0.000000000000000000, -1.000000000000000000, 0.000000000000000000 ) ) ;
#25048=DIRECTION ( 'NONE',  ( -0.000000000000000000, 1.000000000000000000, -0.000000000000000000 ) ) ;
#25049=LINE ( 'NONE', #38011, #13003 ) ;
#25054=PLANE ( 'NONE',  #21046 ) ;
#25082=VECTOR ( 'NONE', #34422, 999.9999999999998863 ) ;
#25095=CARTESIAN_POINT ( 'NONE',  ( 30.00000000000000000, -9.749999999999998224, -13.91584042252958930 ) ) ;
#25127=FACE_OUTER_BOUND ( 'NONE', #26805, .T. ) ;
#25166=CARTESIAN_POINT ( 'NONE',  ( 13.19971406886381793, -9.749999999999998224, -9.306493635776062590 ) ) ;
#25175=CARTESIAN_POINT ( 'NONE',  ( 29.99999999999999645, -3.250000000000000444, -45.99999999999998579 ) ) ;
#25183=VECTOR ( 'NONE', #39272, 1000.000000000000000 ) ;
#25227=ORIENTED_EDGE ( 'NONE', *, *, #29578, .T. ) ;
#25239=CARTESIAN_POINT ( 'NONE',  ( 22.99999999999999645, -9.749999999999998224, -45.99999999999998579 ) ) ;
#25251=EDGE_CURVE ( 'NONE', #7396, #12570, #17221, .T. ) ;
#25287=VECTOR ( 'NONE', #157, 1000.000000000000000 ) ;
#25307=CARTESIAN_POINT ( 'NONE',  ( -10.06976819423596226, 4.478401456986437879, 33.64036950294967454 ) ) ;
#25378=LINE ( 'NONE', #41749, #13992 ) ;
#25405=EDGE_CURVE ( 'NONE', #35361, #24610, #41230, .T. ) ;
#25433=ORIENTED_EDGE ( 'NONE', *, *, #41695, .T. ) ;
#25476=EDGE_CURVE ( 'NONE', #37363, #1431, #33805, .T. ) ;
#25486=AXIS2_PLACEMENT_3D ( 'NONE', #30371, #2222, #20595 ) ;
#25506=AXIS2_PLACEMENT_3D ( 'NONE', #32864, #7558, #20533 ) ;
#25508=EDGE_CURVE ( 'NONE', #31717, #24046, #27117, .T. ) ;
#25510=CARTESIAN_POINT ( 'NONE',  ( 4.257384923554910827, 5.669190722567434726, 44.19375250200204164 ) ) ;
#25525=CARTESIAN_POINT ( 'NONE',  ( -9.808155609017644494, 4.992136686739553575, 34.42174324130925100 ) ) ;
#25557=DIRECTION ( 'NONE',  ( -0.2262442655067633257, 0.000000000000000000, 0.9740705992510528821 ) ) ;
#25565=ORIENTED_EDGE ( 'NONE', *, *, #7268, .T. ) ;
#25581=EDGE_LOOP ( 'NONE', ( #38929, #7122, #34329, #36589, #16701, #7660 ) ) ;
#25586=DIRECTION ( 'NONE',  ( 0.000000000000000000, -0.000000000000000000, -1.000000000000000000 ) ) ;
#25588=CARTESIAN_POINT ( 'NONE',  ( 4.257384923554909051, 7.250000000000000000, 29.19375250200204164 ) ) ;
#25589=EDGE_CURVE ( 'NONE', #41490, #8412, #24235, .T. ) ;
#25594=LINE ( 'NONE', #25175, #5339 ) ;
#25599=DIRECTION ( 'NONE',  ( 0.000000000000000000, 0.000000000000000000, -1.000000000000000000 ) ) ;
#25604=ORIENTED_EDGE ( 'NONE', *, *, #7268, .F. ) ;
#25612=EDGE_CURVE ( 'NONE', #802, #21499, #5430, .T. ) ;
#25704=CARTESIAN_POINT ( 'NONE',  ( -91.72768752788732627, 0.7499999999999997780, -57.39251435732919049 ) ) ;
#25716=DIRECTION ( 'NONE',  ( -1.000000000000000000, 0.000000000000000000, 3.672050975999536074E-16 ) ) ;
#25717=CARTESIAN_POINT ( 'NONE',  ( 9.191929887220489093, 5.970973046099154580, 43.37715118983397389 ) ) ;
#25720=ORIENTED_EDGE ( 'NONE', *, *, #732, .T. ) ;
#25721=VECTOR ( 'NONE', #36890, 1000.000000000000000 ) ;
#25766=CARTESIAN_POINT ( 'NONE',  ( 4.257384923554910827, 7.250000000000000000, 18.45625250200204448 ) ) ;
#25786=DIRECTION ( 'NONE',  ( -0.000000000000000000, 1.000000000000000000, -0.000000000000000000 ) ) ;
#25789=DIRECTION ( 'NONE',  ( 0.000000000000000000, 0.000000000000000000, -1.000000000000000000 ) ) ;
#25854=DIRECTION ( 'NONE',  ( -1.000000000000000000, -0.000000000000000000, -2.102695122396128930E-16 ) ) ;
#25899=LINE ( 'NONE', #35876, #34898 ) ;
#25921=ORIENTED_EDGE ( 'NONE', *, *, #13130, .F. ) ;
#25928=CARTESIAN_POINT ( 'NONE',  ( 9.860324193125613590, 6.050872024979940811, 43.12626573325606216 ) ) ;
#25943=CARTESIAN_POINT ( 'NONE',  ( 0.4112206091368997285, 5.852258295999686055, 43.72431849251835700 ) ) ;
#25945=AXIS2_PLACEMENT_3D ( 'NONE', #10447, #4692, #3848 ) ;
#25961=EDGE_LOOP ( 'NONE', ( #36794, #35372, #40589, #41658, #31601, #479, #14146 ) ) ;
#26018=AXIS2_PLACEMENT_3D ( 'NONE', #14234, #33803, #7861 ) ;
#26038=ORIENTED_EDGE ( 'NONE', *, *, #15246, .T. ) ;
#26054=CIRCLE ( 'NONE', #34870, 6.999999999999992006 ) ;
#26085=AXIS2_PLACEMENT_3D ( 'NONE', #10304, #515, #3294 ) ;
#26111=ORIENTED_EDGE ( 'NONE', *, *, #11993, .T. ) ;
#26127=DIRECTION ( 'NONE',  ( -1.000000000000000000, 0.000000000000000000, 2.768405754343413644E-16 ) ) ;
#26139=VECTOR ( 'NONE', #14270, 1000.000000000000000 ) ;
#26156=CARTESIAN_POINT ( 'NONE',  ( -2.313619569540212861, 6.167084924950640534, 42.71295398355277229 ) ) ;
#26170=DIRECTION ( 'NONE',  ( -1.000000000000000000, -0.000000000000000000, -2.102695122396128930E-16 ) ) ;
#26188=ORIENTED_EDGE ( 'NONE', *, *, #11871, .F. ) ;
#26221=VERTEX_POINT ( 'NONE', #28348 ) ;
#26234=DIRECTION ( 'NONE',  ( -0.000000000000000000, -1.000000000000000000, -0.000000000000000000 ) ) ;
#26268=ORIENTED_EDGE ( 'NONE', *, *, #4821, .T. ) ;
#26272=DIRECTION ( 'NONE',  ( 0.000000000000000000, 0.000000000000000000, 1.000000000000000000 ) ) ;
#26286=FACE_OUTER_BOUND ( 'NONE', #37897, .T. ) ;
#26332=DIRECTION ( 'NONE',  ( 0.000000000000000000, 0.000000000000000000, 1.000000000000000000 ) ) ;
#26334=ORIENTED_EDGE ( 'NONE', *, *, #39180, .T. ) ;
#26345=DIRECTION ( 'NONE',  ( 0.000000000000000000, -0.000000000000000000, -1.000000000000000000 ) ) ;
#26381=ADVANCED_FACE ( 'NONE', ( #6846 ), #10048, .T. ) ;
#26393=EDGE_CURVE ( 'NONE', #24610, #30509, #22598, .T. ) ;
#26431=ADVANCED_FACE ( 'NONE', ( #38016 ), #25054, .F. ) ;
#26459=DIRECTION ( 'NONE',  ( 2.102695122396128930E-16, 0.000000000000000000, -1.000000000000000000 ) ) ;
#26473=EDGE_CURVE ( 'NONE', #569, #14616, #22068, .T. ) ;
#26482=AXIS2_PLACEMENT_3D ( 'NONE', #24543, #8579, #40284 ) ;
#26490=VECTOR ( 'NONE', #16849, 1000.000000000000114 ) ;
#26532=CYLINDRICAL_SURFACE ( 'NONE', #34016, 108.2919410404669378 ) ;
#26548=VERTEX_POINT ( 'NONE', #18670 ) ;
#26565=DIRECTION ( 'NONE',  ( -1.000000000000000000, -0.000000000000000000, -2.102695122396128930E-16 ) ) ;
#26590=B_SPLINE_CURVE_WITH_KNOTS ( 'NONE', 3,
 ( #34896, #18740, #41708, #31702, #6, #32337, #3204, #12986 ),
 .UNSPECIFIED., .F., .F.,
 ( 4, 2, 2, 4 ),
 ( 8.673617379884035472E-19, 0.002163717256739037045, 0.003245575885108555134, 0.004327434513478073223 ),
 .UNSPECIFIED. ) ;
#26641=AXIS2_PLACEMENT_3D ( 'NONE', #21186, #24389, #21603 ) ;
#26642=ADVANCED_FACE ( 'NONE', ( #18874 ), #2708, .T. ) ;
#26651=AXIS2_PLACEMENT_3D ( 'NONE', #13017, #29158, #29797 ) ;
#26664=DIRECTION ( 'NONE',  ( 0.000000000000000000, -1.000000000000000000, 0.000000000000000000 ) ) ;
#26718=AXIS2_PLACEMENT_3D ( 'NONE', #12993, #15992, #25557 ) ;
#26764=AXIS2_PLACEMENT_3D ( 'NONE', #10115, #23080, #35646 ) ;
#26793=AXIS2_PLACEMENT_3D ( 'NONE', #23275, #22654, #26272 ) ;
#26805=EDGE_LOOP ( 'NONE', ( #5962, #4424, #12396, #35732 ) ) ;
#26870=CARTESIAN_POINT ( 'NONE',  ( 14.23381301606215921, 0.7499999999999997780, -13.75869656311284039 ) ) ;
#26913=CARTESIAN_POINT ( 'NONE',  ( 18.38189028304387662, -12.69102426536730377, 34.25298211440382801 ) ) ;
#27001=DIRECTION ( 'NONE',  ( 0.000000000000000000, 0.000000000000000000, -1.000000000000000000 ) ) ;
#27038=PLANE ( 'NONE',  #9643 ) ;
#27059=DIRECTION ( 'NONE',  ( 0.000000000000000000, 0.000000000000000000, -1.000000000000000000 ) ) ;
#27080=( NAMED_UNIT ( * ) PLANE_ANGLE_UNIT ( ) SI_UNIT ( $, .RADIAN. ) );
#27112=ORIENTED_EDGE ( 'NONE', *, *, #20274, .F. ) ;
#27115=ORIENTED_EDGE ( 'NONE', *, *, #20676, .T. ) ;
#27117=CIRCLE ( 'NONE', #19630, 14.99999999999999822 ) ;
#27143=EDGE_CURVE ( 'NONE', #14257, #35065, #23546, .T. ) ;
#27169=EDGE_LOOP ( 'NONE', ( #20349, #23936, #39819, #22556, #27115, #39658 ) ) ;
#27175=ORIENTED_EDGE ( 'NONE', *, *, #20427, .F. ) ;
#27192=VECTOR ( 'NONE', #25035, 1000.000000000000000 ) ;
#27198=DIRECTION ( 'NONE',  ( -1.000000000000000000, -0.000000000000000000, 3.672050975999536567E-16 ) ) ;
#27248=LINE ( 'NONE', #1709, #16626 ) ;
#27293=VERTEX_POINT ( 'NONE', #9254 ) ;
#27304=CARTESIAN_POINT ( 'NONE',  ( 4.257384923554909051, 7.250000000000000000, 29.19375250200204164 ) ) ;
#27374=CARTESIAN_POINT ( 'NONE',  ( 17.89728711128010730, 4.397229927260087656, 35.43499182679077109 ) ) ;
#27385=PLANE ( 'NONE',  #21877 ) ;
#27423=CARTESIAN_POINT ( 'NONE',  ( -33.00000000000001421, 1.750000000000001554, 30.00000000000003908 ) ) ;
#27425=CARTESIAN_POINT ( 'NONE',  ( -8.973752774508733765, -14.84849023317516803, 36.26426228085560410 ) ) ;
#27448=CIRCLE ( 'NONE', #11154, 14.99999999999999822 ) ;
#27454=DIRECTION ( 'NONE',  ( -0.000000000000000000, -1.000000000000000000, -0.000000000000000000 ) ) ;
#27472=DIRECTION ( 'NONE',  ( -0.2262442655067632979, 0.000000000000000000, 0.9740705992510528821 ) ) ;
#27477=AXIS2_PLACEMENT_3D ( 'NONE', #1065, #848, #29974 ) ;
#27478=FACE_OUTER_BOUND ( 'NONE', #28257, .T. ) ;
#27491=EDGE_CURVE ( 'NONE', #223, #12680, #40773, .T. ) ;
#27495=EDGE_CURVE ( 'NONE', #28095, #41095, #36233, .T. ) ;
#27504=CIRCLE ( 'NONE', #37015, 108.2919410404669378 ) ;
#27517=AXIS2_PLACEMENT_3D ( 'NONE', #18611, #24793, #31576 ) ;
#27522=CARTESIAN_POINT ( 'NONE',  ( -7.654597068132072152E-16, 1.750000000000001554, 30.94806650488419919 ) ) ;
#27529=DIRECTION ( 'NONE',  ( 0.000000000000000000, 0.000000000000000000, -1.000000000000000000 ) ) ;
#27544=EDGE_LOOP ( 'NONE', ( #15441, #10720, #623, #6397, #14776, #24516 ) ) ;
#27625=CARTESIAN_POINT ( 'NONE',  ( 0.8967945465527555893, -14.81570784869457214, 43.82048705839584102 ) ) ;
#27633=ORIENTED_EDGE ( 'NONE', *, *, #20676, .F. ) ;
#27637=CARTESIAN_POINT ( 'NONE',  ( 16.03425889574251428, 1.749999999999999778, -46.69170143013996466 ) ) ;
#27674=ADVANCED_FACE ( 'NONE', ( #32218 ), #29017, .T. ) ;
#27692=CARTESIAN_POINT ( 'NONE',  ( -1.827727298698170373E-15, -4.499999999999999112, 36.00000000000000711 ) ) ;
#27724=EDGE_CURVE ( 'NONE', #23286, #22195, #40066, .T. ) ;
#27760=CARTESIAN_POINT ( 'NONE',  ( 30.00000000000000000, 21.91020392607983780, -18.08432671081678578 ) ) ;
#27845=ORIENTED_EDGE ( 'NONE', *, *, #39368, .T. ) ;
#27874=LINE ( 'NONE', #14711, #17277 ) ;
#27925=DIRECTION ( 'NONE',  ( 1.000000000000000000, 0.000000000000000000, 2.102695122396128930E-16 ) ) ;
#27946=VERTEX_POINT ( 'NONE', #28552 ) ;
#27981=CARTESIAN_POINT ( 'NONE',  ( 17.89728711128010730, 5.508031793441324098, 35.43499182679077109 ) ) ;
#28001=DIRECTION ( 'NONE',  ( -0.000000000000000000, 1.000000000000000000, -0.000000000000000000 ) ) ;
#28034=DIRECTION ( 'NONE',  ( 0.000000000000000000, 0.000000000000000000, -1.000000000000000000 ) ) ;
#28066=CIRCLE ( 'NONE', #2273, 10.99999999999998934 ) ;
#28089=ORIENTED_EDGE ( 'NONE', *, *, #905, .F. ) ;
#28095=VERTEX_POINT ( 'NONE', #38967 ) ;
#28096=CIRCLE ( 'NONE', #15240, 9.999999999999973355 ) ;
#28123=CYLINDRICAL_SURFACE ( 'NONE', #40251, 10.73749999999999716 ) ;
#28131=PLANE ( 'NONE',  #13200 ) ;
#28137=ORIENTED_EDGE ( 'NONE', *, *, #30609, .F. ) ;
#28161=ORIENTED_EDGE ( 'NONE', *, *, #38937, .T. ) ;
#28175=DIRECTION ( 'NONE',  ( 0.000000000000000000, 0.000000000000000000, 1.000000000000000000 ) ) ;
#28177=CARTESIAN_POINT ( 'NONE',  ( 17.89728711128010730, -4.500000000000000000, 40.00000000000002842 ) ) ;
#28203=ORIENTED_EDGE ( 'NONE', *, *, #20182, .T. ) ;
#28211=CARTESIAN_POINT ( 'NONE',  ( 4.257384923554910827, 7.250000000000000000, 44.19375250200204164 ) ) ;
#28213=CARTESIAN_POINT ( 'NONE',  ( 33.00000000000001421, 1.750000000000001554, 32.19375250200203453 ) ) ;
#28222=ORIENTED_EDGE ( 'NONE', *, *, #17119, .F. ) ;
#28229=CARTESIAN_POINT ( 'NONE',  ( 4.257384923554909939, -19.75000000000000000, 23.69375250200204874 ) ) ;
#28248=LINE ( 'NONE', #5710, #3624 ) ;
#28249=DIRECTION ( 'NONE',  ( -0.000000000000000000, 1.000000000000000000, -0.000000000000000000 ) ) ;
#28256=VERTEX_POINT ( 'NONE', #24082 ) ;
#28257=EDGE_LOOP ( 'NONE', ( #3508, #6078, #6643, #26038 ) ) ;
#28263=CARTESIAN_POINT ( 'NONE',  ( 5.689851406550298307, 5.690848806005884164, 44.14229661063782828 ) ) ;
#28268=ADVANCED_FACE ( 'NONE', ( #7908 ), #20457, .T. ) ;
#28302=ORIENTED_EDGE ( 'NONE', *, *, #41755, .T. ) ;
#28348=CARTESIAN_POINT ( 'NONE',  ( -10.63967459768254642, -10.75000000000000000, 30.94806650488419564 ) ) ;
#28409=ORIENTED_EDGE ( 'NONE', *, *, #30821, .T. ) ;
#28412=ORIENTED_EDGE ( 'NONE', *, *, #26473, .T. ) ;
#28428=ADVANCED_FACE ( 'NONE', ( #21695 ), #5121, .T. ) ;
#28552=CARTESIAN_POINT ( 'NONE',  ( 16.03425889574251428, 0.7499999999999997780, -46.69170143013996466 ) ) ;
#28558=DIRECTION ( 'NONE',  ( -0.000000000000000000, 1.000000000000000000, -0.000000000000000000 ) ) ;
#28577=EDGE_CURVE ( 'NONE', #18534, #35066, #34260, .T. ) ;
#28618=EDGE_LOOP ( 'NONE', ( #10420, #18375, #40901, #17753 ) ) ;
#28635=VECTOR ( 'NONE', #17826, 1000.000000000000000 ) ;
#28670=VERTEX_POINT ( 'NONE', #29495 ) ;
#28680=ORIENTED_EDGE ( 'NONE', *, *, #31341, .T. ) ;
#28717=ADVANCED_FACE ( 'NONE', ( #7176 ), #26532, .T. ) ;
#28775=CARTESIAN_POINT ( 'NONE',  ( 4.257384923554909051, 7.250000000000000000, 29.19375250200204164 ) ) ;
#28822=CIRCLE ( 'NONE', #10487, 10.99999999999998934 ) ;
#28829=VERTEX_POINT ( 'NONE', #20981 ) ;
#28853=DIRECTION ( 'NONE',  ( -2.102695122396129176E-16, 0.000000000000000000, 1.000000000000000000 ) ) ;
#28876=CARTESIAN_POINT ( 'NONE',  ( -12.28065031820330155, 0.7499999999999997780, 16.19629439043522012 ) ) ;
#28878=DIRECTION ( 'NONE',  ( 0.000000000000000000, 0.000000000000000000, -1.000000000000000000 ) ) ;
#28884=ORIENTED_EDGE ( 'NONE', *, *, #41434, .T. ) ;
#28885=ORIENTED_EDGE ( 'NONE', *, *, #15246, .F. ) ;
#28890=FACE_OUTER_BOUND ( 'NONE', #1851, .T. ) ;
#28893=CARTESIAN_POINT ( 'NONE',  ( 18.95432338025397812, 1.750000000000001554, 32.19375250200202743 ) ) ;
#28907=CARTESIAN_POINT ( 'NONE',  ( 3.280145919556070044, 5.679155502329209071, 44.16982272867637249 ) ) ;
#28943=CIRCLE ( 'NONE', #29616, 15.00000000000000000 ) ;
#28953=DIRECTION ( 'NONE',  ( -1.000000000000000000, -0.000000000000000000, -2.102695122396128930E-16 ) ) ;
#29017=PLANE ( 'NONE',  #6134 ) ;
#29027=FACE_OUTER_BOUND ( 'NONE', #4772, .T. ) ;
#29034=ORIENTED_EDGE ( 'NONE', *, *, #7232, .F. ) ;
#29045=VERTEX_POINT ( 'NONE', #27981 ) ;
#29057=EDGE_CURVE ( 'NONE', #15754, #37673, #1437, .T. ) ;
#29062=DIRECTION ( 'NONE',  ( -0.000000000000000000, 1.000000000000000000, -0.000000000000000000 ) ) ;
#29095=CARTESIAN_POINT ( 'NONE',  ( 16.03425889574250363, -9.749999999999998224, -46.69170143013996466 ) ) ;
#29110=CARTESIAN_POINT ( 'NONE',  ( -9.295555791501751486, 5.607854746313242877, 35.63702243816140225 ) ) ;
#29129=ORIENTED_EDGE ( 'NONE', *, *, #14639, .F. ) ;
#29149=DIRECTION ( 'NONE',  ( 0.000000000000000000, 0.000000000000000000, -1.000000000000000000 ) ) ;
#29158=DIRECTION ( 'NONE',  ( -0.000000000000000000, 1.000000000000000000, -0.000000000000000000 ) ) ;
#29181=EDGE_CURVE ( 'NONE', #28829, #16560, #14338, .T. ) ;
#29182=VERTEX_POINT ( 'NONE', #15018 ) ;
#29184=DIRECTION ( 'NONE',  ( -0.000000000000000000, 1.000000000000000000, -0.000000000000000000 ) ) ;
#29227=VERTEX_POINT ( 'NONE', #9691 ) ;
#29230=EDGE_LOOP ( 'NONE', ( #40703, #32551, #34032, #26111 ) ) ;
#29238=CARTESIAN_POINT ( 'NONE',  ( -91.72768752788732627, -3.250000000000000444, -57.39251435732919049 ) ) ;
#29301=CARTESIAN_POINT ( 'NONE',  ( 33.00000000000001421, -4.500000000000000000, 40.00000000000002842 ) ) ;
#29427=DIRECTION ( 'NONE',  ( -2.542075073846521157E-16, -0.000000000000000000, -1.000000000000000000 ) ) ;
#29462=VECTOR ( 'NONE', #34785, 1000.000000000000000 ) ;
#29470=ADVANCED_BREP_SHAPE_REPRESENTATION ( '', ( #22626, #40442 ), #16010 ) ;
#29492=EDGE_CURVE ( 'NONE', #41395, #30509, #35394, .T. ) ;
#29495=CARTESIAN_POINT ( 'NONE',  ( -26.68952268848979870, 1.750000000000001554, 29.19375250200205230 ) ) ;
#29531=EDGE_CURVE ( 'NONE', #30663, #35066, #41072, .T. ) ;
#29532=CARTESIAN_POINT ( 'NONE',  ( 11.79574205785023366, -15.28867464124770059, 42.18168139380896520 ) ) ;
#29539=EDGE_CURVE ( 'NONE', #35992, #8731, #5548, .T. ) ;
#29561=CIRCLE ( 'NONE', #4471, 15.00000000000000000 ) ;
#29578=EDGE_CURVE ( 'NONE', #5338, #16560, #11509, .T. ) ;
#29613=CARTESIAN_POINT ( 'NONE',  ( -11.21606888246744127, 0.7499999999999997780, 29.19375250200204519 ) ) ;
#29616=AXIS2_PLACEMENT_3D ( 'NONE', #34641, #8482, #24667 ) ;
#29628=EDGE_CURVE ( 'NONE', #31717, #36959, #1939, .T. ) ;
#29682=ADVANCED_FACE ( 'NONE', ( #25127 ), #34481, .T. ) ;
#29686=ADVANCED_FACE ( 'NONE', ( #41288 ), #12133, .F. ) ;
#29691=DIRECTION ( 'NONE',  ( 1.000000000000000000, 0.000000000000000000, -2.768405754343413644E-16 ) ) ;
#29797=DIRECTION ( 'NONE',  ( 0.000000000000000000, 0.000000000000000000, 1.000000000000000000 ) ) ;
#29851=DIRECTION ( 'NONE',  ( 1.000000000000000000, 0.000000000000000000, 2.102695122396128930E-16 ) ) ;
#29870=AXIS2_PLACEMENT_3D ( 'NONE', #33003, #41756, #19408 ) ;
#29884=FACE_OUTER_BOUND ( 'NONE', #40985, .T. ) ;
#29952=DIRECTION ( 'NONE',  ( 0.000000000000000000, 0.000000000000000000, -1.000000000000000000 ) ) ;
#29955=CARTESIAN_POINT ( 'NONE',  ( 17.29116825269524682, -14.99555005906381489, 36.65099875778255978 ) ) ;
#29959=AXIS2_PLACEMENT_3D ( 'NONE', #24714, #37676, #11929 ) ;
#29974=DIRECTION ( 'NONE',  ( 2.102695122396128930E-16, 0.000000000000000000, -1.000000000000000000 ) ) ;
#30021=AXIS2_PLACEMENT_3D ( 'NONE', #40802, #1474, #11050 ) ;
#30047=VECTOR ( 'NONE', #26234, 1000.000000000000000 ) ;
#30073=AXIS2_PLACEMENT_3D ( 'NONE', #30735, #1598, #14578 ) ;
#30089=ORIENTED_EDGE ( 'NONE', *, *, #8404, .F. ) ;
#30097=EDGE_CURVE ( 'NONE', #41070, #35065, #23159, .T. ) ;
#30170=CARTESIAN_POINT ( 'NONE',  ( 13.85158599686961267, -15.47832887086968867, 40.72984191034792900 ) ) ;
#30181=CYLINDRICAL_SURFACE ( 'NONE', #26018, 6.999999999999992006 ) ;
#30185=CARTESIAN_POINT ( 'NONE',  ( -11.21606888246744127, -9.749999999999998224, 29.19375250200204519 ) ) ;
#30209=VERTEX_POINT ( 'NONE', #15132 ) ;
#30215=CARTESIAN_POINT ( 'NONE',  ( 4.257384923554909051, -19.75000000000000000, 14.19375250200204341 ) ) ;
#30256=CARTESIAN_POINT ( 'NONE',  ( -17.89728711128011440, -10.75000000000000000, 32.19375250200205585 ) ) ;
#30265=VECTOR ( 'NONE', #1667, 1000.000000000000000 ) ;
#30284=EDGE_CURVE ( 'NONE', #8624, #41395, #26590, .T. ) ;
#30312=ADVANCED_FACE ( 'NONE', ( #14341 ), #14766, .T. ) ;
#30369=EDGE_CURVE ( 'NONE', #8731, #22296, #24337, .T. ) ;
#30371=CARTESIAN_POINT ( 'NONE',  ( 4.257384923554909051, -10.75000000000000000, 29.19375250200204164 ) ) ;
#30452=CYLINDRICAL_SURFACE ( 'NONE', #8052, 10.00000000000000178 ) ;
#30463=ORIENTED_EDGE ( 'NONE', *, *, #31833, .T. ) ;
#30481=AXIS2_PLACEMENT_3D ( 'NONE', #16551, #23346, #26332 ) ;
#30501=EDGE_CURVE ( 'NONE', #3004, #7535, #33861, .T. ) ;
#30509=VERTEX_POINT ( 'NONE', #33479 ) ;
#30544=AXIS2_PLACEMENT_3D ( 'NONE', #9515, #34410, #5270 ) ;
#30549=ORIENTED_EDGE ( 'NONE', *, *, #39509, .F. ) ;
#30574=EDGE_LOOP ( 'NONE', ( #40919, #17180, #17755, #16092, #12786, #206, #39343, #15465, #25604, #11880, #1157 ) ) ;
#30603=DIRECTION ( 'NONE',  ( -0.2645837230171119159, 0.000000000000000000, -0.9643627188534427130 ) ) ;
#30609=EDGE_CURVE ( 'NONE', #8476, #2310, #35153, .T. ) ;
#30634=EDGE_CURVE ( 'NONE', #19770, #41715, #11975, .T. ) ;
#30652=EDGE_CURVE ( 'NONE', #21343, #35361, #25594, .T. ) ;
#30661=LINE ( 'NONE', #1320, #22408 ) ;
#30663=VERTEX_POINT ( 'NONE', #21969 ) ;
#30677=FACE_OUTER_BOUND ( 'NONE', #24825, .T. ) ;
#30696=FACE_OUTER_BOUND ( 'NONE', #20216, .T. ) ;
#30721=VERTEX_POINT ( 'NONE', #7060 ) ;
#30730=CARTESIAN_POINT ( 'NONE',  ( 33.00000000000001421, -4.499999999999999112, 36.00000000000002842 ) ) ;
#30735=CARTESIAN_POINT ( 'NONE',  ( 4.257384923554909051, -9.749999999999998224, 29.19375250200204164 ) ) ;
#30736=CARTESIAN_POINT ( 'NONE',  ( 29.99999999999999645, -3.250000000000000444, -45.99999999999998579 ) ) ;
#30747=CIRCLE ( 'NONE', #5609, 4.000000000000031086 ) ;
#30782=LINE ( 'NONE', #1644, #21743 ) ;
#30785=PLANE ( 'NONE',  #37115 ) ;
#30799=FACE_OUTER_BOUND ( 'NONE', #8785, .T. ) ;
#30813=FACE_OUTER_BOUND ( 'NONE', #11003, .T. ) ;
#30816=DIRECTION ( 'NONE',  ( -0.000000000000000000, 1.000000000000000000, -0.000000000000000000 ) ) ;
#30821=EDGE_CURVE ( 'NONE', #33538, #36380, #12814, .T. ) ;
#30837=ORIENTED_EDGE ( 'NONE', *, *, #22005, .F. ) ;
#30843=CIRCLE ( 'NONE', #15932, 10.73749999999999716 ) ;
#30870=ORIENTED_EDGE ( 'NONE', *, *, #5928, .F. ) ;
#30875=DIRECTION ( 'NONE',  ( -0.2262442655067632979, 0.000000000000000000, 0.9740705992510528821 ) ) ;
#30888=ORIENTED_EDGE ( 'NONE', *, *, #41662, .T. ) ;
#30893=ADVANCED_FACE ( 'NONE', ( #27478 ), #30452, .T. ) ;
#30897=EDGE_LOOP ( 'NONE', ( #15405, #28222, #23813, #9541 ) ) ;
#30909=FACE_OUTER_BOUND ( 'NONE', #24966, .T. ) ;
#30912=DIRECTION ( 'NONE',  ( 0.000000000000000000, -0.000000000000000000, 1.000000000000000000 ) ) ;
#30938=ORIENTED_EDGE ( 'NONE', *, *, #4957, .T. ) ;
#30943=EDGE_CURVE ( 'NONE', #21705, #34231, #31649, .T. ) ;
#30958=CYLINDRICAL_SURFACE ( 'NONE', #3725, 10.73749999999999716 ) ;
#30960=PLANE ( 'NONE',  #13814 ) ;
#30983=EDGE_LOOP ( 'NONE', ( #29129, #28412, #20421, #6797 ) ) ;
#31026=DIRECTION ( 'NONE',  ( 0.000000000000000000, -1.000000000000000000, 0.000000000000000000 ) ) ;
#31027=CARTESIAN_POINT ( 'NONE',  ( -10.06856782476305590, -13.48118709369469492, 33.64427118030894803 ) ) ;
#31078=ORIENTED_EDGE ( 'NONE', *, *, #34435, .F. ) ;
#31116=EDGE_CURVE ( 'NONE', #8412, #27946, #22306, .T. ) ;
#31174=DIRECTION ( 'NONE',  ( -0.000000000000000000, 1.000000000000000000, -0.000000000000000000 ) ) ;
#31189=ORIENTED_EDGE ( 'NONE', *, *, #16818, .T. ) ;
#31191=AXIS2_PLACEMENT_3D ( 'NONE', #9234, #31355, #8812 ) ;
#31211=CYLINDRICAL_SURFACE ( 'NONE', #11846, 9.999999999999994671 ) ;
#31227=CARTESIAN_POINT ( 'NONE',  ( 2.323739122872637175, -14.70923867967206888, 44.10015179151258025 ) ) ;
#31239=CARTESIAN_POINT ( 'NONE',  ( 23.34627465269464253, -5.749999999999999112, -52.99143003003683816 ) ) ;
#31274=DIRECTION ( 'NONE',  ( -3.469446951953623557E-16, 0.000000000000000000, 1.000000000000000000 ) ) ;
#31278=AXIS2_PLACEMENT_3D ( 'NONE', #4093, #13668, #914 ) ;
#31341=EDGE_CURVE ( 'NONE', #23286, #30209, #36735, .T. ) ;
#31349=CARTESIAN_POINT ( 'NONE',  ( 17.89728711128010730, -13.39722992726008854, 35.43499182679077109 ) ) ;
#31355=DIRECTION ( 'NONE',  ( 3.672050975999536074E-16, -0.000000000000000000, 1.000000000000000000 ) ) ;
#31356=DIRECTION ( 'NONE',  ( -0.08163352362547934837, 0.000000000000000000, -0.9966624141706601492 ) ) ;
#31397=ORIENTED_EDGE ( 'NONE', *, *, #32887, .T. ) ;
#31410=ADVANCED_FACE ( 'NONE', ( #33549 ), #33115, .T. ) ;
#31419=DIRECTION ( 'NONE',  ( -0.000000000000000000, 1.000000000000000000, -0.000000000000000000 ) ) ;
#31420=CARTESIAN_POINT ( 'NONE',  ( -2.668805347656625298E-15, -4.500000000000000000, 40.00000000000002132 ) ) ;
#31440=ORIENTED_EDGE ( 'NONE', *, *, #25612, .F. ) ;
#31446=ORIENTED_EDGE ( 'NONE', *, *, #32766, .F. ) ;
#31453=CARTESIAN_POINT ( 'NONE',  ( 14.65257870790896355, 6.510049746086139955, 40.03135401722945375 ) ) ;
#31455=EDGE_CURVE ( 'NONE', #39665, #24287, #4000, .T. ) ;
#31484=ORIENTED_EDGE ( 'NONE', *, *, #13609, .F. ) ;
#31490=CARTESIAN_POINT ( 'NONE',  ( 23.34627465269464253, -3.250000000000000444, -52.99143003003683816 ) ) ;
#31563=AXIS2_PLACEMENT_3D ( 'NONE', #36212, #40261, #33237 ) ;
#31576=DIRECTION ( 'NONE',  ( -2.102695122396129176E-16, 0.000000000000000000, 1.000000000000000000 ) ) ;
#31589=EDGE_LOOP ( 'NONE', ( #36905, #21721, #39774, #30089, #26268, #7491, #16147, #27175, #7700, #36009, #28203 ) ) ;
#31601=ORIENTED_EDGE ( 'NONE', *, *, #25508, .T. ) ;
#31649=LINE ( 'NONE', #10895, #38621 ) ;
#31686=DIRECTION ( 'NONE',  ( -1.000000000000000000, -0.000000000000000000, -2.102695122396128930E-16 ) ) ;
#31693=ORIENTED_EDGE ( 'NONE', *, *, #684, .F. ) ;
#31702=CARTESIAN_POINT ( 'NONE',  ( 18.64829610662276949, 3.050960375449419448, 33.43445880657997549 ) ) ;
#31710=DIRECTION ( 'NONE',  ( 0.000000000000000000, 0.000000000000000000, -1.000000000000000000 ) ) ;
#31717=VERTEX_POINT ( 'NONE', #15659 ) ;
#31797=CARTESIAN_POINT ( 'NONE',  ( 22.99999999999999645, 0.7499999999999997780, -45.99999999999998579 ) ) ;
#31816=ORIENTED_EDGE ( 'NONE', *, *, #11613, .T. ) ;
#31833=EDGE_CURVE ( 'NONE', #30721, #17500, #19602, .T. ) ;
#31870=CARTESIAN_POINT ( 'NONE',  ( 17.89728711128010730, 5.508031793441324098, 35.43499182679077109 ) ) ;
#31904=ORIENTED_EDGE ( 'NONE', *, *, #41010, .T. ) ;
#31918=CYLINDRICAL_SURFACE ( 'NONE', #32145, 4.000000000000017764 ) ;
#31927=ORIENTED_EDGE ( 'NONE', *, *, #30943, .F. ) ;
#31998=DIRECTION ( 'NONE',  ( -0.000000000000000000, -1.000000000000000000, -0.000000000000000000 ) ) ;
#32015=LINE ( 'NONE', #2881, #34106 ) ;
#32035=DIRECTION ( 'NONE',  ( -0.000000000000000000, 1.000000000000000000, -0.000000000000000000 ) ) ;
#32048=DIRECTION ( 'NONE',  ( -1.000000000000000000, -0.000000000000000000, -2.102695122396128930E-16 ) ) ;
#32053=DIRECTION ( 'NONE',  ( 0.000000000000000000, -1.000000000000000000, 0.000000000000000000 ) ) ;
#32054=VECTOR ( 'NONE', #29427, 1000.000000000000000 ) ;
#32061=APPLICATION_CONTEXT ( 'automotive_design' ) ;
#32065=DIRECTION ( 'NONE',  ( -0.9643627188534427130, 0.000000000000000000, 0.2645837230171117493 ) ) ;
#32103=SHAPE_REPRESENTATION ( 'Aluminum Fixing Part', ( #40442 ), #16010 ) ;
#32104=EDGE_CURVE ( 'NONE', #21499, #802, #4678, .T. ) ;
#32120=ORIENTED_EDGE ( 'NONE', *, *, #22740, .T. ) ;
#32126=DIRECTION ( 'NONE',  ( -0.000000000000000000, 1.000000000000000000, -0.000000000000000000 ) ) ;
#32144=VERTEX_POINT ( 'NONE', #18998 ) ;
#32145=AXIS2_PLACEMENT_3D ( 'NONE', #214, #13195, #39133 ) ;
#32171=CARTESIAN_POINT ( 'NONE',  ( 19.25738492355490550, 7.250000000000000000, 29.19375250200203453 ) ) ;
#32182=ORIENTED_EDGE ( 'NONE', *, *, #34435, .T. ) ;
#32218=FACE_OUTER_BOUND ( 'NONE', #528, .T. ) ;
#32241=DIRECTION ( 'NONE',  ( 0.000000000000000000, 0.000000000000000000, -1.000000000000000000 ) ) ;
#32274=DIRECTION ( 'NONE',  ( -0.000000000000000000, -1.000000000000000000, -0.000000000000000000 ) ) ;
#32315=CARTESIAN_POINT ( 'NONE',  ( -6.597596034333014003, 6.496367707564395744, 39.55742414453274591 ) ) ;
#32336=EDGE_LOOP ( 'NONE', ( #25921, #11362 ) ) ;
#32337=CARTESIAN_POINT ( 'NONE',  ( 18.85346025669424108, 2.302299922872062865, 32.66119954658682900 ) ) ;
#32396=LINE ( 'NONE', #41775, #38345 ) ;
#32480=ORIENTED_EDGE ( 'NONE', *, *, #4294, .T. ) ;
#32518=CARTESIAN_POINT ( 'NONE',  ( -4.778401075125691122, 6.441207554884578634, 41.17682173525715683 ) ) ;
#32534=ORIENTED_EDGE ( 'NONE', *, *, #20274, .T. ) ;
#32538=ORIENTED_EDGE ( 'NONE', *, *, #2837, .F. ) ;
#32543=FACE_OUTER_BOUND ( 'NONE', #19357, .T. ) ;
#32551=ORIENTED_EDGE ( 'NONE', *, *, #26393, .F. ) ;
#32625=AXIS2_PLACEMENT_3D ( 'NONE', #36024, #39419, #3084 ) ;
#32704=ORIENTED_EDGE ( 'NONE', *, *, #22389, .T. ) ;
#32723=CARTESIAN_POINT ( 'NONE',  ( -9.090079023779228606, 5.776958475262540915, 36.05404750004154835 ) ) ;
#32751=VERTEX_POINT ( 'NONE', #23588 ) ;
#32758=AXIS2_PLACEMENT_3D ( 'NONE', #27304, #26664, #40480 ) ;
#32766=EDGE_CURVE ( 'NONE', #32851, #41070, #17202, .T. ) ;
#32773=FACE_OUTER_BOUND ( 'NONE', #3969, .T. ) ;
#32800=DIRECTION ( 'NONE',  ( 0.000000000000000000, 0.000000000000000000, 1.000000000000000000 ) ) ;
#32804=DIRECTION ( 'NONE',  ( -0.08163352362547934837, 0.000000000000000000, -0.9966624141706601492 ) ) ;
#32828=CARTESIAN_POINT ( 'NONE',  ( -10.74261507644509450, 1.749999999999999778, 29.19375250200204519 ) ) ;
#32837=CARTESIAN_POINT ( 'NONE',  ( 23.34627465269464253, -9.749999999999998224, -52.99143003003683816 ) ) ;
#32851=VERTEX_POINT ( 'NONE', #38010 ) ;
#32855=CARTESIAN_POINT ( 'NONE',  ( 4.257384923554910827, -19.75000000000000000, 44.19375250200204164 ) ) ;
#32864=CARTESIAN_POINT ( 'NONE',  ( 4.257384923554909051, -10.75000000000000000, 29.19375250200204164 ) ) ;
#32887=EDGE_CURVE ( 'NONE', #36959, #1431, #40997, .T. ) ;
#32905=CARTESIAN_POINT ( 'NONE',  ( 13.19971406886381615, 0.7499999999999997780, -9.306493635776055484 ) ) ;
#32919=CARTESIAN_POINT ( 'NONE',  ( 30.00000000000000000, -9.749999999999998224, -13.91584042252958930 ) ) ;
#32927=AXIS2_PLACEMENT_3D ( 'NONE', #14258, #1490, #14467 ) ;
#32946=FACE_BOUND ( 'NONE', #34746, .T. ) ;
#32963=VECTOR ( 'NONE', #12496, 1000.000000000000000 ) ;
#33003=CARTESIAN_POINT ( 'NONE',  ( -91.72768752788732627, -5.749999999999999112, -57.39251435732919049 ) ) ;
#33026=( LENGTH_UNIT ( ) NAMED_UNIT ( * ) SI_UNIT ( .MILLI., .METRE. ) );
#33063=ORIENTED_EDGE ( 'NONE', *, *, #16109, .T. ) ;
#33070=ORIENTED_EDGE ( 'NONE', *, *, #27495, .F. ) ;
#33088=LINE ( 'NONE', #36499, #4305 ) ;
#33115=CYLINDRICAL_SURFACE ( 'NONE', #15556, 14.99999999999999822 ) ;
#33119=ORIENTED_EDGE ( 'NONE', *, *, #12617, .F. ) ;
#33123=ORIENTED_EDGE ( 'NONE', *, *, #15968, .F. ) ;
#33130=LINE ( 'NONE', #9387, #34591 ) ;
#33156=DIRECTION ( 'NONE',  ( -0.000000000000000000, 1.000000000000000000, -0.000000000000000000 ) ) ;
#33170=VERTEX_POINT ( 'NONE', #35860 ) ;
#33175=VECTOR ( 'NONE', #15397, 1000.000000000000114 ) ;
#33237=DIRECTION ( 'NONE',  ( 0.000000000000000000, 0.000000000000000000, 1.000000000000000000 ) ) ;
#33264=DIRECTION ( 'NONE',  ( -0.000000000000000000, 1.000000000000000000, -0.000000000000000000 ) ) ;
#33273=ORIENTED_EDGE ( 'NONE', *, *, #41695, .F. ) ;
#33277=VERTEX_POINT ( 'NONE', #20964 ) ;
#33315=ORIENTED_EDGE ( 'NONE', *, *, #37533, .F. ) ;
#33344=CARTESIAN_POINT ( 'NONE',  ( 30.00000000000002132, -3.250000000000000444, -18.08432671081678578 ) ) ;
#33357=CARTESIAN_POINT ( 'NONE',  ( 12.99284412668524880, -15.41362446690534505, 41.39301592953864883 ) ) ;
#33382=EDGE_LOOP ( 'NONE', ( #5014, #35141, #10211, #39499, #1646, #6388 ) ) ;
#33406=LINE ( 'NONE', #4270, #34146 ) ;
#33420=AXIS2_PLACEMENT_3D ( 'NONE', #36572, #1884, #4664 ) ;
#33439=VERTEX_POINT ( 'NONE', #8823 ) ;
#33479=CARTESIAN_POINT ( 'NONE',  ( 19.25738492355488773, 1.749999999999999778, 29.19375250200203453 ) ) ;
#33507=CIRCLE ( 'NONE', #15175, 10.73749999999999716 ) ;
#33538=VERTEX_POINT ( 'NONE', #5419 ) ;
#33544=ADVANCED_FACE ( 'NONE', ( #24580 ), #30958, .F. ) ;
#33549=FACE_OUTER_BOUND ( 'NONE', #25961, .T. ) ;
#33577=ADVANCED_FACE ( 'NONE', ( #34355 ), #12008, .T. ) ;
#33580=LINE ( 'NONE', #23800, #36104 ) ;
#33672=CARTESIAN_POINT ( 'NONE',  ( 33.00000000000001421, -4.500000000000000000, 40.00000000000002842 ) ) ;
#33691=CARTESIAN_POINT ( 'NONE',  ( -72.11291920797204114, -5.749999999999999112, 14.09998371085514179 ) ) ;
#33710=ORIENTED_EDGE ( 'NONE', *, *, #16898, .T. ) ;
#33717=DIRECTION ( 'NONE',  ( 2.768405754343413644E-16, 0.000000000000000000, 1.000000000000000000 ) ) ;
#33718=CARTESIAN_POINT ( 'NONE',  ( 18.15916614181498545, -13.07070140576124473, 34.83626390038371312 ) ) ;
#33759=CARTESIAN_POINT ( 'NONE',  ( -12.28065031820330155, -9.749999999999998224, 16.19629439043522012 ) ) ;
#33761=CARTESIAN_POINT ( 'NONE',  ( 4.257384923554909051, 7.250000000000000000, 29.19375250200204164 ) ) ;
#33803=DIRECTION ( 'NONE',  ( -0.000000000000000000, -1.000000000000000000, -0.000000000000000000 ) ) ;
#33805=LINE ( 'NONE', #24441, #3341 ) ;
#33812=ORIENTED_EDGE ( 'NONE', *, *, #25476, .T. ) ;
#33817=VERTEX_POINT ( 'NONE', #16885 ) ;
#33861=CIRCLE ( 'NONE', #26482, 5.499999999999991118 ) ;
#33895=CARTESIAN_POINT ( 'NONE',  ( 4.257384923554909939, 0.8500000000000017542, 23.69375250200204519 ) ) ;
#33899=ORIENTED_EDGE ( 'NONE', *, *, #37884, .F. ) ;
#33901=CARTESIAN_POINT ( 'NONE',  ( -73.17652798666306069, -3.250000000000000444, 10.22331041471092483 ) ) ;
#33926=VECTOR ( 'NONE', #13311, 1000.000000000000000 ) ;
#33937=ADVANCED_FACE ( 'NONE', ( #30696 ), #1968, .F. ) ;
#33978=FACE_OUTER_BOUND ( 'NONE', #19371, .T. ) ;
#33988=CIRCLE ( 'NONE', #39400, 6.999999999999992006 ) ;
#34016=AXIS2_PLACEMENT_3D ( 'NONE', #9745, #6746, #35685 ) ;
#34032=ORIENTED_EDGE ( 'NONE', *, *, #25405, .F. ) ;
#34051=DIRECTION ( 'NONE',  ( -0.000000000000000000, 1.000000000000000000, -0.000000000000000000 ) ) ;
#34058=CARTESIAN_POINT ( 'NONE',  ( -17.89728711128011440, -4.500000000000000000, 40.00000000000001421 ) ) ;
#34076=VECTOR ( 'NONE', #31419, 1000.000000000000000 ) ;
#34083=EDGE_LOOP ( 'NONE', ( #40388, #33070, #1, #5241, #31078, #29034, #3509, #33063 ) ) ;
#34095=CARTESIAN_POINT ( 'NONE',  ( -91.72768752788732627, -10.75000000000000000, -57.39251435732919049 ) ) ;
#34106=VECTOR ( 'NONE', #6493, 1000.000000000000114 ) ;
#34146=VECTOR ( 'NONE', #14691, 1000.000000000000000 ) ;
#34180=ORIENTED_EDGE ( 'NONE', *, *, #3221, .F. ) ;
#34182=CIRCLE ( 'NONE', #4178, 9.999999999999987566 ) ;
#34213=CARTESIAN_POINT ( 'NONE',  ( -9.805985683824957277, -13.99565755907026876, 34.42765945797622607 ) ) ;
#34216=CARTESIAN_POINT ( 'NONE',  ( 4.257384923554910827, 7.250000000000000000, 44.19375250200204164 ) ) ;
#34220=LINE ( 'NONE', #14870, #14422 ) ;
#34231=VERTEX_POINT ( 'NONE', #20187 ) ;
#34260=LINE ( 'NONE', #4187, #25183 ) ;
#34285=EDGE_CURVE ( 'NONE', #7535, #11862, #19393, .T. ) ;
#34319=DIRECTION ( 'NONE',  ( 0.000000000000000000, -1.000000000000000000, 0.000000000000000000 ) ) ;
#34322=DIRECTION ( 'NONE',  ( 0.000000000000000000, 1.000000000000000000, 0.000000000000000000 ) ) ;
#34329=ORIENTED_EDGE ( 'NONE', *, *, #30943, .T. ) ;
#34355=FACE_OUTER_BOUND ( 'NONE', #27544, .T. ) ;
#34410=DIRECTION ( 'NONE',  ( -1.000000000000000000, -0.000000000000000000, -2.102695122396128930E-16 ) ) ;
#34422=DIRECTION ( 'NONE',  ( -0.08163352362547934837, -0.000000000000000000, -0.9966624141706601492 ) ) ;
#34435=EDGE_CURVE ( 'NONE', #34649, #29182, #39957, .T. ) ;
#34481=PLANE ( 'NONE',  #29959 ) ;
#34517=FACE_BOUND ( 'NONE', #7749, .T. ) ;
#34538=ORIENTED_EDGE ( 'NONE', *, *, #25508, .F. ) ;
#34540=DIRECTION ( 'NONE',  ( 0.000000000000000000, -1.000000000000000000, 0.000000000000000000 ) ) ;
#34541=CARTESIAN_POINT ( 'NONE',  ( 32.99999999999999289, -10.75000000000000000, -45.99999999999999289 ) ) ;
#34560=DIRECTION ( 'NONE',  ( -3.154042683594197586E-16, 0.000000000000000000, 1.000000000000000000 ) ) ;
#34584=ORIENTED_EDGE ( 'NONE', *, *, #37233, .T. ) ;
#34591=VECTOR ( 'NONE', #12575, 1000.000000000000114 ) ;
#34631=EDGE_CURVE ( 'NONE', #13500, #13232, #29561, .T. ) ;
#34641=CARTESIAN_POINT ( 'NONE',  ( 4.257384923554909051, -3.250000000000000444, 29.19375250200204164 ) ) ;
#34649=VERTEX_POINT ( 'NONE', #2501 ) ;
#34655=FACE_OUTER_BOUND ( 'NONE', #18425, .T. ) ;
#34659=VECTOR ( 'NONE', #4597, 1000.000000000000000 ) ;
#34672=EDGE_CURVE ( 'NONE', #39544, #4123, #21639, .T. ) ;
#34701=ORIENTED_EDGE ( 'NONE', *, *, #338, .T. ) ;
#34715=CARTESIAN_POINT ( 'NONE',  ( 4.257384923554909051, 7.250000000000000000, 29.19375250200204164 ) ) ;
#34734=CARTESIAN_POINT ( 'NONE',  ( 23.34627465269464253, -5.749999999999999112, -52.99143003003683816 ) ) ;
#34746=EDGE_LOOP ( 'NONE', ( #15366, #36347 ) ) ;
#34784=DIRECTION ( 'NONE',  ( 0.000000000000000000, -1.000000000000000000, 0.000000000000000000 ) ) ;
#34785=DIRECTION ( 'NONE',  ( 2.102695122396128930E-16, 0.000000000000000000, -1.000000000000000000 ) ) ;
#34802=DIRECTION ( 'NONE',  ( -2.102695122396128190E-16, 0.000000000000000000, 1.000000000000000000 ) ) ;
#34809=CARTESIAN_POINT ( 'NONE',  ( -1.027389493830889017E-15, -10.75000000000000000, 32.19375250200202743 ) ) ;
#34827=CARTESIAN_POINT ( 'NONE',  ( 30.00000000000000000, 21.91020392607983780, -18.08432671081678578 ) ) ;
#34828=DIRECTION ( 'NONE',  ( 0.000000000000000000, 0.000000000000000000, -1.000000000000000000 ) ) ;
#34865=CIRCLE ( 'NONE', #6342, 10.99999999999998934 ) ;
#34870=AXIS2_PLACEMENT_3D ( 'NONE', #31797, #15235, #24601 ) ;
#34877=VECTOR ( 'NONE', #24030, 1000.000000000000000 ) ;
#34896=CARTESIAN_POINT ( 'NONE',  ( 17.89728711128010730, 4.397229927260087656, 35.43499182679077109 ) ) ;
#34898=VECTOR ( 'NONE', #32274, 1000.000000000000000 ) ;
#34910=VERTEX_POINT ( 'NONE', #19505 ) ;
#34984=DIRECTION ( 'NONE',  ( -1.000000000000000000, -0.000000000000000000, 3.672050975999536567E-16 ) ) ;
#35010=VERTEX_POINT ( 'NONE', #31349 ) ;
#35018=LINE ( 'NONE', #28211, #27192 ) ;
#35019=EDGE_LOOP ( 'NONE', ( #10249, #27845 ) ) ;
#35020=EDGE_CURVE ( 'NONE', #39425, #24819, #14643, .T. ) ;
#35065=VERTEX_POINT ( 'NONE', #5827 ) ;
#35066=VERTEX_POINT ( 'NONE', #34541 ) ;
#35071=CARTESIAN_POINT ( 'NONE',  ( 11.78318312939863155, 6.287241406411228972, 42.18929554591962017 ) ) ;
#35098=ORIENTED_EDGE ( 'NONE', *, *, #20992, .T. ) ;
#35102=EDGE_LOOP ( 'NONE', ( #41498, #4720, #41699, #24729 ) ) ;
#35114=ADVANCED_FACE ( 'NONE', ( #6030 ), #3460, .F. ) ;
#35141=ORIENTED_EDGE ( 'NONE', *, *, #31116, .T. ) ;
#35153=LINE ( 'NONE', #12612, #39279 ) ;
#35163=ORIENTED_EDGE ( 'NONE', *, *, #20144, .T. ) ;
#35201=CYLINDRICAL_SURFACE ( 'NONE', #9817, 14.99999999999999822 ) ;
#35225=ADVANCED_FACE ( 'NONE', ( #2841 ), #6453, .F. ) ;
#35244=PLANE ( 'NONE',  #24783 ) ;
#35262=CARTESIAN_POINT ( 'NONE',  ( 17.89728711128010730, -4.500000000000000000, 40.00000000000002842 ) ) ;
#35294=CARTESIAN_POINT ( 'NONE',  ( 3.771639164433389535, 5.669190722567432950, 44.19375250200204874 ) ) ;
#35310=CARTESIAN_POINT ( 'NONE',  ( -91.72768752788732627, -3.250000000000000444, -57.39251435732919049 ) ) ;
#35318=VERTEX_POINT ( 'NONE', #30256 ) ;
#35327=DIRECTION ( 'NONE',  ( 0.000000000000000000, -1.000000000000000000, 0.000000000000000000 ) ) ;
#35332=ORIENTED_EDGE ( 'NONE', *, *, #6114, .F. ) ;
#35344=DIRECTION ( 'NONE',  ( -1.000000000000000000, 0.000000000000000000, 3.672050975999536567E-16 ) ) ;
#35357=PLANE ( 'NONE',  #39784 ) ;
#35361=VERTEX_POINT ( 'NONE', #37479 ) ;
#35372=ORIENTED_EDGE ( 'NONE', *, *, #12620, .T. ) ;
#35394=CIRCLE ( 'NONE', #37433, 15.00000000000000000 ) ;
#35401=DIRECTION ( 'NONE',  ( -1.000000000000000000, 0.000000000000000000, 3.672050975999536567E-16 ) ) ;
#35416=CARTESIAN_POINT ( 'NONE',  ( 13.19971406886381615, -5.749999999999999112, -9.306493635776055484 ) ) ;
#35436=EDGE_LOOP ( 'NONE', ( #24157, #40021, #36420, #5611 ) ) ;
#35440=CIRCLE ( 'NONE', #17108, 9.999999999999987566 ) ;
#35471=CARTESIAN_POINT ( 'NONE',  ( 4.257384923554909051, -19.75000000000000000, 29.19375250200204164 ) ) ;
#35491=VECTOR ( 'NONE', #40894, 1000.000000000000114 ) ;
#35517=AXIS2_PLACEMENT_3D ( 'NONE', #1675, #4454, #27001 ) ;
#35544=EDGE_LOOP ( 'NONE', ( #35163, #11599, #23400, #2734, #32534, #20008, #34538, #31816, #25433, #40814, #16388, #9970 ) ) ;
#35589=LINE ( 'NONE', #29613, #30047 ) ;
#35636=ORIENTED_EDGE ( 'NONE', *, *, #3833, .F. ) ;
#35646=DIRECTION ( 'NONE',  ( 0.000000000000000000, 0.000000000000000000, 1.000000000000000000 ) ) ;
#35653=CARTESIAN_POINT ( 'NONE',  ( 13.04894127963215666, 1.750000000000001554, -46.98814490019994139 ) ) ;
#35685=DIRECTION ( 'NONE',  ( 0.000000000000000000, 0.000000000000000000, 1.000000000000000000 ) ) ;
#35719=CARTESIAN_POINT ( 'NONE',  ( -5.540078435796097267, 6.489926879127195569, 40.56252941885252739 ) ) ;
#35728=CYLINDRICAL_SURFACE ( 'NONE', #15087, 10.99999999999998934 ) ;
#35732=ORIENTED_EDGE ( 'NONE', *, *, #19271, .T. ) ;
#35786=EDGE_CURVE ( 'NONE', #35992, #21705, #41848, .T. ) ;
#35829=DIRECTION ( 'NONE',  ( -0.000000000000000000, -1.000000000000000000, -0.000000000000000000 ) ) ;
#35844=PLANE ( 'NONE',  #15895 ) ;
#35860=CARTESIAN_POINT ( 'NONE',  ( -10.74261507644508740, 0.7499999999999997780, 29.19375250200204519 ) ) ;
#35876=CARTESIAN_POINT ( 'NONE',  ( -33.00000000000001421, 1.750000000000001554, 30.00000000000003908 ) ) ;
#35877=VERTEX_POINT ( 'NONE', #5774 ) ;
#35917=CARTESIAN_POINT ( 'NONE',  ( -9.653604622060775853, 5.215829120183355094, 34.82245567039050371 ) ) ;
#35939=ORIENTED_EDGE ( 'NONE', *, *, #21618, .T. ) ;
#35976=LINE ( 'NONE', #248, #2268 ) ;
#35992=VERTEX_POINT ( 'NONE', #11227 ) ;
#36009=ORIENTED_EDGE ( 'NONE', *, *, #37533, .T. ) ;
#36024=CARTESIAN_POINT ( 'NONE',  ( -17.89728711128011440, -4.500000000000000000, 40.00000000000001421 ) ) ;
#36070=PLANE ( 'NONE',  #3620 ) ;
#36104=VECTOR ( 'NONE', #21017, 1000.000000000000114 ) ;
#36110=CARTESIAN_POINT ( 'NONE',  ( 9.757384923554903722, 0.8500000000000013101, 29.19375250200204164 ) ) ;
#36155=ADVANCED_FACE ( 'NONE', ( #33978, #4836 ), #30785, .T. ) ;
#36190=CARTESIAN_POINT ( 'NONE',  ( -26.68952268848979870, -3.250000000000000444, 29.19375250200205230 ) ) ;
#36201=VERTEX_POINT ( 'NONE', #28213 ) ;
#36206=CARTESIAN_POINT ( 'NONE',  ( 7.651048906156353802, 7.250000000000000000, 14.58269351323625251 ) ) ;
#36212=CARTESIAN_POINT ( 'NONE',  ( 33.00000000000001421, -4.500000000000000000, 40.00000000000002842 ) ) ;
#36233=LINE ( 'NONE', #6887, #14305 ) ;
#36239=CIRCLE ( 'NONE', #17915, 10.00000000000000178 ) ;
#36340=CARTESIAN_POINT ( 'NONE',  ( 17.89728711128010730, -14.50803179344132410, 35.43499182679077109 ) ) ;
#36347=ORIENTED_EDGE ( 'NONE', *, *, #30501, .F. ) ;
#36380=VERTEX_POINT ( 'NONE', #2480 ) ;
#36420=ORIENTED_EDGE ( 'NONE', *, *, #12699, .F. ) ;
#36454=CARTESIAN_POINT ( 'NONE',  ( 23.34627465269464253, -3.250000000000000444, -52.99143003003683816 ) ) ;
#36477=CARTESIAN_POINT ( 'NONE',  ( 18.03526480546840105, -13.24251363533436354, 35.13344879104447216 ) ) ;
#36499=CARTESIAN_POINT ( 'NONE',  ( -4.771500470052752946E-15, -4.500000000000000000, 50.00000000000001421 ) ) ;
#36532=ORIENTED_EDGE ( 'NONE', *, *, #20511, .F. ) ;
#36535=CARTESIAN_POINT ( 'NONE',  ( -17.89728711128011795, 1.750000000000001554, 49.99999999999998579 ) ) ;
#36553=CARTESIAN_POINT ( 'NONE',  ( 7.124026683171984509, -14.77278659301236630, 43.93473567553544257 ) ) ;
#36572=CARTESIAN_POINT ( 'NONE',  ( 22.99999999999999645, -10.75000000000000000, -45.99999999999998579 ) ) ;
#36589=ORIENTED_EDGE ( 'NONE', *, *, #41010, .F. ) ;
#36650=DIRECTION ( 'NONE',  ( 1.000000000000000000, 0.000000000000000000, 0.000000000000000000 ) ) ;
#36682=EDGE_CURVE ( 'NONE', #12679, #22195, #28943, .T. ) ;
#36702=EDGE_CURVE ( 'NONE', #38940, #15754, #37628, .T. ) ;
#36706=CYLINDRICAL_SURFACE ( 'NONE', #38420, 108.2919410404669378 ) ;
#36735=LINE ( 'NONE', #32905, #10786 ) ;
#36740=CARTESIAN_POINT ( 'NONE',  ( -11.21606888246744482, -3.250000000000000444, 29.19375250200204519 ) ) ;
#36745=AXIS2_PLACEMENT_3D ( 'NONE', #2459, #34784, #15870 ) ;
#36750=EDGE_LOOP ( 'NONE', ( #42031, #38502, #21148, #788, #10221 ) ) ;
#36764=CARTESIAN_POINT ( 'NONE',  ( 17.89728711128010730, 7.250000000000000000, 35.43499182679077109 ) ) ;
#36790=ORIENTED_EDGE ( 'NONE', *, *, #25251, .T. ) ;
#36794=ORIENTED_EDGE ( 'NONE', *, *, #8037, .F. ) ;
#36795=DIRECTION ( 'NONE',  ( -0.9643627188534427130, 0.000000000000000000, 0.2645837230171117493 ) ) ;
#36856=ORIENTED_EDGE ( 'NONE', *, *, #13130, .T. ) ;
#36859=EDGE_CURVE ( 'NONE', #27293, #28256, #37174, .T. ) ;
#36861=AXIS2_PLACEMENT_3D ( 'NONE', #29301, #19956, #171 ) ;
#36884=LINE ( 'NONE', #27522, #16034 ) ;
#36890=DIRECTION ( 'NONE',  ( 0.9643627188534427130, 0.000000000000000000, -0.2645837230171117493 ) ) ;
#36905=ORIENTED_EDGE ( 'NONE', *, *, #4311, .T. ) ;
#36928=FACE_OUTER_BOUND ( 'NONE', #34083, .T. ) ;
#36955=DIRECTION ( 'NONE',  ( 0.000000000000000000, 0.000000000000000000, -1.000000000000000000 ) ) ;
#36959=VERTEX_POINT ( 'NONE', #24405 ) ;
#36978=CARTESIAN_POINT ( 'NONE',  ( -11.21606888246744127, -9.749999999999998224, 29.19375250200204519 ) ) ;
#37015=AXIS2_PLACEMENT_3D ( 'NONE', #16121, #29062, #10562 ) ;
#37031=CARTESIAN_POINT ( 'NONE',  ( 29.99999999999999645, -10.75000000000000000, -45.99999999999998579 ) ) ;
#37033=FACE_OUTER_BOUND ( 'NONE', #17237, .T. ) ;
#37100=DIRECTION ( 'NONE',  ( 0.2262442655067633257, 0.000000000000000000, -0.9740705992510528821 ) ) ;
#37115=AXIS2_PLACEMENT_3D ( 'NONE', #1647, #24411, #37377 ) ;
#37121=EDGE_LOOP ( 'NONE', ( #8638, #37364, #9705, #40237 ) ) ;
#37173=DIRECTION ( 'NONE',  ( 0.9740705992510528821, -0.000000000000000000, 0.2262442655067633257 ) ) ;
#37174=LINE ( 'NONE', #36535, #3823 ) ;
#37177=ORIENTED_EDGE ( 'NONE', *, *, #30652, .T. ) ;
#37206=CARTESIAN_POINT ( 'NONE',  ( -9.082706494909455586, -14.77117114956869592, 36.05632303781640502 ) ) ;
#37233=EDGE_CURVE ( 'NONE', #15664, #11308, #20629, .T. ) ;
#37325=VERTEX_POINT ( 'NONE', #32855 ) ;
#37331=ADVANCED_FACE ( 'NONE', ( #26286 ), #35844, .T. ) ;
#37363=VERTEX_POINT ( 'NONE', #19890 ) ;
#37364=ORIENTED_EDGE ( 'NONE', *, *, #12617, .T. ) ;
#37377=DIRECTION ( 'NONE',  ( -2.102695122396128930E-16, 0.000000000000000000, 1.000000000000000000 ) ) ;
#37409=CARTESIAN_POINT ( 'NONE',  ( -6.921836208682301539, -15.47785305164596004, 39.20696469929084316 ) ) ;
#37433=AXIS2_PLACEMENT_3D ( 'NONE', #11977, #34322, #18366 ) ;
#37479=CARTESIAN_POINT ( 'NONE',  ( 30.00000000000001776, -3.250000000000000444, 29.19375250200203098 ) ) ;
#37506=ORIENTED_EDGE ( 'NONE', *, *, #5150, .T. ) ;
#37507=AXIS2_PLACEMENT_3D ( 'NONE', #12874, #25854, #2667 ) ;
#37524=CARTESIAN_POINT ( 'NONE',  ( -26.68952268848979870, -3.250000000000000444, 29.19375250200205230 ) ) ;
#37533=EDGE_CURVE ( 'NONE', #5666, #35010, #5605, .T. ) ;
#37614=CARTESIAN_POINT ( 'NONE',  ( -10.18218683828283666, -13.19693995854222379, 33.26054558596090516 ) ) ;
#37618=DIRECTION ( 'NONE',  ( -1.000000000000000000, -0.000000000000000000, -2.102695122396128930E-16 ) ) ;
#37620=CARTESIAN_POINT ( 'NONE',  ( -4.771500470052749002E-15, -4.500000000000000000, 50.00000000000000000 ) ) ;
#37627=EDGE_LOOP ( 'NONE', ( #10474, #1112, #2571, #4293, #10958, #30463, #19112, #8261, #11461, #16769, #17165, #3143, #39982, #31904, #9545, #17699 ) ) ;
#37628=LINE ( 'NONE', #31239, #6565 ) ;
#37673=VERTEX_POINT ( 'NONE', #3860 ) ;
#37676=DIRECTION ( 'NONE',  ( -0.9966624141706600382, 0.000000000000000000, 0.08163352362547933450 ) ) ;
#37785=ORIENTED_EDGE ( 'NONE', *, *, #14671, .T. ) ;
#37832=ORIENTED_EDGE ( 'NONE', *, *, #27143, .T. ) ;
#37851=CARTESIAN_POINT ( 'NONE',  ( 23.34627465269464253, -9.749999999999998224, -52.99143003003683816 ) ) ;
#37869=LINE ( 'NONE', #8727, #3169 ) ;
#37884=EDGE_CURVE ( 'NONE', #14616, #39665, #36239, .T. ) ;
#37897=EDGE_LOOP ( 'NONE', ( #9277, #9173, #15778, #14456, #18074 ) ) ;
#37964=CARTESIAN_POINT ( 'NONE',  ( 4.257384923554909051, 0.8500000000000017542, 34.69375250200203453 ) ) ;
#38010=CARTESIAN_POINT ( 'NONE',  ( 4.257384923554910827, 0.8500000000000009770, 18.45625250200204448 ) ) ;
#38011=CARTESIAN_POINT ( 'NONE',  ( 23.34627465269464253, -9.749999999999998224, -52.99143003003683816 ) ) ;
#38016=FACE_OUTER_BOUND ( 'NONE', #5824, .T. ) ;
#38019=ORIENTED_EDGE ( 'NONE', *, *, #34631, .T. ) ;
#38035=DIRECTION ( 'NONE',  ( -1.000000000000000000, -0.000000000000000000, -2.102695122396128930E-16 ) ) ;
#38092=CARTESIAN_POINT ( 'NONE',  ( -26.68952268848979870, -5.749999999999999112, 29.19375250200205230 ) ) ;
#38136=DIRECTION ( 'NONE',  ( 2.768405754343413644E-16, 0.000000000000000000, 1.000000000000000000 ) ) ;
#38144=ADVANCED_FACE ( 'NONE', ( #32946, #6587 ), #22955, .T. ) ;
#38152=DIRECTION ( 'NONE',  ( 0.000000000000000000, 1.000000000000000000, 0.000000000000000000 ) ) ;
#38165=LINE ( 'NONE', #18609, #40152 ) ;
#38170=EDGE_CURVE ( 'NONE', #17500, #32144, #24234, .T. ) ;
#38184=CARTESIAN_POINT ( 'NONE',  ( -17.89728711128011795, -10.75000000000000000, 49.99999999999998579 ) ) ;
#38201=DIRECTION ( 'NONE',  ( -1.000000000000000000, -0.000000000000000000, -2.102695122396128930E-16 ) ) ;
#38204=DIRECTION ( 'NONE',  ( 0.000000000000000000, -1.000000000000000000, 0.000000000000000000 ) ) ;
#38256=CARTESIAN_POINT ( 'NONE',  ( 7.805100899383003110, 5.833159988962552056, 43.77259587910655370 ) ) ;
#38345=VECTOR ( 'NONE', #32804, 999.9999999999998863 ) ;
#38369=VECTOR ( 'NONE', #40783, 1000.000000000000000 ) ;
#38399=CARTESIAN_POINT ( 'NONE',  ( -91.72768752788732627, -3.250000000000000444, -57.39251435732919049 ) ) ;
#38400=CARTESIAN_POINT ( 'NONE',  ( 4.257384923554909051, 7.250000000000000000, 29.19375250200204164 ) ) ;
#38406=ORIENTED_EDGE ( 'NONE', *, *, #24056, .T. ) ;
#38414=DIRECTION ( 'NONE',  ( 0.000000000000000000, 1.000000000000000000, 0.000000000000000000 ) ) ;
#38420=AXIS2_PLACEMENT_3D ( 'NONE', #4381, #4163, #7570 ) ;
#38474=CARTESIAN_POINT ( 'NONE',  ( 12.99709304830720136, 6.416992383093250929, 41.40601189719725284 ) ) ;
#38476=EDGE_CURVE ( 'NONE', #11300, #37325, #27448, .T. ) ;
#38483=DIRECTION ( 'NONE',  ( 0.000000000000000000, -1.000000000000000000, 0.000000000000000000 ) ) ;
#38485=CARTESIAN_POINT ( 'NONE',  ( 23.34627465269464253, 0.7499999999999997780, -52.99143003003683816 ) ) ;
#38489=CARTESIAN_POINT ( 'NONE',  ( -10.23457012397624410, 4.045242672364334879, 33.06917214921114834 ) ) ;
#38502=ORIENTED_EDGE ( 'NONE', *, *, #9872, .T. ) ;
#38520=FACE_OUTER_BOUND ( 'NONE', #35019, .T. ) ;
#38607=DIRECTION ( 'NONE',  ( 0.000000000000000000, -1.000000000000000000, 0.000000000000000000 ) ) ;
#38621=VECTOR ( 'NONE', #28249, 1000.000000000000000 ) ;
#38652=VECTOR ( 'NONE', #25048, 1000.000000000000000 ) ;
#38696=CARTESIAN_POINT ( 'NONE',  ( -8.637089462929189665, 6.054629030046592142, 36.87170610838806084 ) ) ;
#38723=CIRCLE ( 'NONE', #5444, 10.73749999999999716 ) ;
#38743=DIRECTION ( 'NONE',  ( 0.000000000000000000, 0.000000000000000000, -1.000000000000000000 ) ) ;
#38778=DIRECTION ( 'NONE',  ( 0.000000000000000000, 0.000000000000000000, -1.000000000000000000 ) ) ;
#38818=FACE_OUTER_BOUND ( 'NONE', #30983, .T. ) ;
#38831=DIRECTION ( 'NONE',  ( 0.000000000000000000, 1.000000000000000000, 0.000000000000000000 ) ) ;
#38881=LINE ( 'NONE', #13142, #16484 ) ;
#38887=VECTOR ( 'NONE', #35344, 1000.000000000000000 ) ;
#38929=ORIENTED_EDGE ( 'NONE', *, *, #3747, .T. ) ;
#38937=EDGE_CURVE ( 'NONE', #35318, #223, #41597, .T. ) ;
#38939=ADVANCED_FACE ( 'NONE', ( #21815 ), #35201, .T. ) ;
#38940=VERTEX_POINT ( 'NONE', #35416 ) ;
#38967=CARTESIAN_POINT ( 'NONE',  ( 29.99999999999999645, -5.749999999999999112, -45.99999999999998579 ) ) ;
#39026=SHAPE_DEFINITION_REPRESENTATION ( #4776, #32103 ) ;
#39107=CARTESIAN_POINT ( 'NONE',  ( -10.46692563697871314, 3.269548650761419317, 32.15430906845504921 ) ) ;
#39128=VERTEX_POINT ( 'NONE', #21602 ) ;
#39133=DIRECTION ( 'NONE',  ( -2.102695122396128190E-16, 0.000000000000000000, 1.000000000000000000 ) ) ;
#39151=LINE ( 'NONE', #10033, #38887 ) ;
#39172=EDGE_CURVE ( 'NONE', #37363, #2310, #5038, .T. ) ;
#39180=EDGE_CURVE ( 'NONE', #41673, #36201, #15215, .T. ) ;
#39224=VERTEX_POINT ( 'NONE', #32837 ) ;
#39233=DIRECTION ( 'NONE',  ( -0.000000000000000000, 1.000000000000000000, -0.000000000000000000 ) ) ;
#39238=ORIENTED_EDGE ( 'NONE', *, *, #9207, .F. ) ;
#39253=DIRECTION ( 'NONE',  ( -1.000000000000000000, -0.000000000000000000, -2.102695122396128930E-16 ) ) ;
#39272=DIRECTION ( 'NONE',  ( -2.542075073846521157E-16, -0.000000000000000000, -1.000000000000000000 ) ) ;
#39279=VECTOR ( 'NONE', #28558, 1000.000000000000000 ) ;
#39326=PLANE ( 'NONE',  #12164 ) ;
#39343=ORIENTED_EDGE ( 'NONE', *, *, #31116, .F. ) ;
#39368=EDGE_CURVE ( 'NONE', #32851, #14257, #30843, .T. ) ;
#39377=DIRECTION ( 'NONE',  ( -1.000000000000000000, 0.000000000000000000, 3.672050975999536567E-16 ) ) ;
#39391=CARTESIAN_POINT ( 'NONE',  ( 22.99999999999999645, 1.750000000000001554, -45.99999999999998579 ) ) ;
#39400=AXIS2_PLACEMENT_3D ( 'NONE', #25239, #38204, #9068 ) ;
#39419=DIRECTION ( 'NONE',  ( -1.000000000000000000, -0.000000000000000000, -2.102695122396128930E-16 ) ) ;
#39425=VERTEX_POINT ( 'NONE', #8881 ) ;
#39499=ORIENTED_EDGE ( 'NONE', *, *, #10088, .F. ) ;
#39509=EDGE_CURVE ( 'NONE', #19770, #28095, #5731, .T. ) ;
#39522=ADVANCED_FACE ( 'NONE', ( #21638 ), #35244, .T. ) ;
#39544=VERTEX_POINT ( 'NONE', #9090 ) ;
#39548=VECTOR ( 'NONE', #7062, 1000.000000000000000 ) ;
#39561=ORIENTED_EDGE ( 'NONE', *, *, #39180, .F. ) ;
#39599=VERTEX_POINT ( 'NONE', #22478 ) ;
#39603=AXIS2_PLACEMENT_3D ( 'NONE', #6726, #6098, #19079 ) ;
#39625=CARTESIAN_POINT ( 'NONE',  ( 18.95432338025397456, -10.75000000000000000, 32.19375250200202743 ) ) ;
#39630=CLOSED_SHELL ( 'NONE', ( #33544, #10172, #30312, #5606, #21530, #26642, #33577, #21523, #2007, #18070, #19830, #26381, #11669, #24888, #24404, #37331, #4009, #15329, #27674, #13801, #7315, #22974, #14517, #10799, #6969, #29686, #10816, #21244, #28268, #15400, #36155, #13984, #39522, #12353, #9756, #3043, #2073, #20213, #30893, #33937, #28717, #35114, #15994, #11351, #28428, #29682, #39976, #38939, #38144, #31410, #35225, #22045, #5682, #10820, #11966, #26431, #17634 ) ) ;
#39658=ORIENTED_EDGE ( 'NONE', *, *, #15968, .T. ) ;
#39665=VERTEX_POINT ( 'NONE', #780 ) ;
#39716=EDGE_LOOP ( 'NONE', ( #13723, #7827, #2559, #36856 ) ) ;
#39747=CARTESIAN_POINT ( 'NONE',  ( 12.69825749791893621, -15.38500454582616683, 41.59858831224365616 ) ) ;
#39768=CIRCLE ( 'NONE', #3740, 9.999999999999980460 ) ;
#39774=ORIENTED_EDGE ( 'NONE', *, *, #38476, .F. ) ;
#39781=ORIENTED_EDGE ( 'NONE', *, *, #40486, .T. ) ;
#39784=AXIS2_PLACEMENT_3D ( 'NONE', #8988, #12605, #25586 ) ;
#39819=ORIENTED_EDGE ( 'NONE', *, *, #8231, .F. ) ;
#39869=ORIENTED_EDGE ( 'NONE', *, *, #38476, .T. ) ;
#39904=CARTESIAN_POINT ( 'NONE',  ( 4.257384923554909051, 7.250000000000000000, 39.93125250200203880 ) ) ;
#39927=EDGE_LOOP ( 'NONE', ( #32120, #14403, #17192, #19162, #37177, #2569, #7935, #31927 ) ) ;
#39957=LINE ( 'NONE', #11038, #30265 ) ;
#39976=ADVANCED_FACE ( 'NONE', ( #8002 ), #28131, .T. ) ;
#39982=ORIENTED_EDGE ( 'NONE', *, *, #10088, .T. ) ;
#40021=ORIENTED_EDGE ( 'NONE', *, *, #2370, .F. ) ;
#40031=AXIS2_PLACEMENT_3D ( 'NONE', #36110, #35327, #26345 ) ;
#40066=LINE ( 'NONE', #36454, #14273 ) ;
#40077=CARTESIAN_POINT ( 'NONE',  ( -91.72768752788732627, 1.750000000000001554, -57.39251435732919049 ) ) ;
#40147=DIRECTION ( 'NONE',  ( -0.9643627188534427130, 0.000000000000000000, 0.2645837230171117493 ) ) ;
#40152=VECTOR ( 'NONE', #24998, 1000.000000000000000 ) ;
#40204=VECTOR ( 'NONE', #15216, 1000.000000000000000 ) ;
#40237=ORIENTED_EDGE ( 'NONE', *, *, #4294, .F. ) ;
#40251=AXIS2_PLACEMENT_3D ( 'NONE', #34715, #5583, #18555 ) ;
#40261=DIRECTION ( 'NONE',  ( -1.000000000000000000, -0.000000000000000000, -2.102695122396128930E-16 ) ) ;
#40284=DIRECTION ( 'NONE',  ( 0.000000000000000000, 0.000000000000000000, -1.000000000000000000 ) ) ;
#40299=PRODUCT_DEFINITION ( 'UNKNOWN', '', #13259, #6310 ) ;
#40358=CARTESIAN_POINT ( 'NONE',  ( 23.34627465269464253, 0.7499999999999997780, -52.99143003003683816 ) ) ;
#40388=ORIENTED_EDGE ( 'NONE', *, *, #41662, .F. ) ;
#40392=CARTESIAN_POINT ( 'NONE',  ( 30.00000000000001776, -3.250000000000000444, 29.19375250200203098 ) ) ;
#40396=LINE ( 'NONE', #34216, #17228 ) ;
#40403=ORIENTED_EDGE ( 'NONE', *, *, #35786, .F. ) ;
#40421=CARTESIAN_POINT ( 'NONE',  ( -91.72768752788732627, -5.749999999999999112, -57.39251435732919049 ) ) ;
#40432=CARTESIAN_POINT ( 'NONE',  ( 22.99999999999999645, -10.75000000000000000, -45.99999999999998579 ) ) ;
#40442=AXIS2_PLACEMENT_3D ( 'NONE', #11131, #24112, #36650 ) ;
#40457=DIRECTION ( 'NONE',  ( -0.000000000000000000, -1.000000000000000000, -0.000000000000000000 ) ) ;
#40480=DIRECTION ( 'NONE',  ( 0.000000000000000000, 0.000000000000000000, -1.000000000000000000 ) ) ;
#40486=EDGE_CURVE ( 'NONE', #12570, #2310, #32396, .T. ) ;
#40589=ORIENTED_EDGE ( 'NONE', *, *, #41755, .F. ) ;
#40591=FACE_OUTER_BOUND ( 'NONE', #30897, .T. ) ;
#40650=EDGE_CURVE ( 'NONE', #17635, #26548, #3037, .T. ) ;
#40703=ORIENTED_EDGE ( 'NONE', *, *, #1501, .F. ) ;
#40749=FACE_OUTER_BOUND ( 'NONE', #41608, .T. ) ;
#40768=DIRECTION ( 'NONE',  ( 0.000000000000000000, 0.000000000000000000, 1.000000000000000000 ) ) ;
#40773=CIRCLE ( 'NONE', #32625, 10.99999999999998934 ) ;
#40783=DIRECTION ( 'NONE',  ( -1.000000000000000000, -0.000000000000000000, 3.672050975999536567E-16 ) ) ;
#40799=PLANE ( 'NONE',  #9035 ) ;
#40802=CARTESIAN_POINT ( 'NONE',  ( -17.89728711128011440, -4.500000000000000000, 40.00000000000001421 ) ) ;
#40806=AXIS2_PLACEMENT_3D ( 'NONE', #1108, #17483, #670 ) ;
#40814=ORIENTED_EDGE ( 'NONE', *, *, #14150, .T. ) ;
#40862=CARTESIAN_POINT ( 'NONE',  ( -10.74261507644508740, 7.250000000000000000, 29.19375250200204874 ) ) ;
#40887=VECTOR ( 'NONE', #21554, 1000.000000000000000 ) ;
#40894=DIRECTION ( 'NONE',  ( 0.9643627188534427130, 0.000000000000000000, -0.2645837230171119159 ) ) ;
#40901=ORIENTED_EDGE ( 'NONE', *, *, #5928, .T. ) ;
#40902=VECTOR ( 'NONE', #16866, 1000.000000000000000 ) ;
#40919=ORIENTED_EDGE ( 'NONE', *, *, #21470, .F. ) ;
#40922=DIRECTION ( 'NONE',  ( -3.672050975999536074E-16, 0.000000000000000000, -1.000000000000000000 ) ) ;
#40932=CARTESIAN_POINT ( 'NONE',  ( 33.00000000000001421, -4.500000000000000000, 50.00000000000002842 ) ) ;
#40946=LINE ( 'NONE', #8825, #20619 ) ;
#40984=VECTOR ( 'NONE', #34984, 1000.000000000000000 ) ;
#40985=EDGE_LOOP ( 'NONE', ( #6612, #5728, #14088, #5858 ) ) ;
#40997=LINE ( 'NONE', #21846, #38369 ) ;
#40998=DIRECTION ( 'NONE',  ( -0.2262442655067632979, 0.000000000000000000, 0.9740705992510528821 ) ) ;
#41010=EDGE_CURVE ( 'NONE', #15662, #34231, #11861, .T. ) ;
#41033=CARTESIAN_POINT ( 'NONE',  ( -33.00000000000002132, -4.500000000000000000, 44.00000000000004263 ) ) ;
#41070=VERTEX_POINT ( 'NONE', #25766 ) ;
#41072=LINE ( 'NONE', #24707, #4830 ) ;
#41080=DIRECTION ( 'NONE',  ( 0.000000000000000000, -1.000000000000000000, 0.000000000000000000 ) ) ;
#41095=VERTEX_POINT ( 'NONE', #21934 ) ;
#41189=ORIENTED_EDGE ( 'NONE', *, *, #7141, .F. ) ;
#41192=ORIENTED_EDGE ( 'NONE', *, *, #30821, .F. ) ;
#41230=LINE ( 'NONE', #40392, #42094 ) ;
#41242=ORIENTED_EDGE ( 'NONE', *, *, #29492, .T. ) ;
#41247=CARTESIAN_POINT ( 'NONE',  ( 16.10492761103993686, 6.400234005401329362, 38.42205234425481564 ) ) ;
#41288=FACE_OUTER_BOUND ( 'NONE', #10775, .T. ) ;
#41320=CARTESIAN_POINT ( 'NONE',  ( -91.72768752788732627, 1.749999999999999778, -57.39251435732919049 ) ) ;
#41348=FACE_OUTER_BOUND ( 'NONE', #29230, .T. ) ;
#41365=EDGE_CURVE ( 'NONE', #37325, #11300, #13933, .T. ) ;
#41395=VERTEX_POINT ( 'NONE', #28893 ) ;
#41396=ORIENTED_EDGE ( 'NONE', *, *, #32887, .F. ) ;
#41416=VERTEX_POINT ( 'NONE', #29095 ) ;
#41430=DIRECTION ( 'NONE',  ( 0.000000000000000000, 0.000000000000000000, 1.000000000000000000 ) ) ;
#41434=EDGE_CURVE ( 'NONE', #2398, #29045, #13290, .T. ) ;
#41475=CARTESIAN_POINT ( 'NONE',  ( -10.63967459768254820, 1.750000000000001554, 30.94806650488419564 ) ) ;
#41490=VERTEX_POINT ( 'NONE', #2952 ) ;
#41498=ORIENTED_EDGE ( 'NONE', *, *, #39368, .F. ) ;
#41509=VECTOR ( 'NONE', #30875, 1000.000000000000114 ) ;
#41541=DIRECTION ( 'NONE',  ( 0.000000000000000000, 0.000000000000000000, 1.000000000000000000 ) ) ;
#41558=ORIENTED_EDGE ( 'NONE', *, *, #12925, .F. ) ;
#41597=LINE ( 'NONE', #38184, #29462 ) ;
#41598=AXIS2_PLACEMENT_3D ( 'NONE', #41320, #25786, #9622 ) ;
#41599=CARTESIAN_POINT ( 'NONE',  ( 22.99999999999999645, 1.750000000000001554, -45.99999999999998579 ) ) ;
#41608=EDGE_LOOP ( 'NONE', ( #21459, #14825, #24856 ) ) ;
#41628=AXIS2_PLACEMENT_3D ( 'NONE', #12469, #38414, #9279 ) ;
#41658=ORIENTED_EDGE ( 'NONE', *, *, #29628, .F. ) ;
#41662=EDGE_CURVE ( 'NONE', #41095, #33439, #8814, .T. ) ;
#41673=VERTEX_POINT ( 'NONE', #40932 ) ;
#41684=CARTESIAN_POINT ( 'NONE',  ( -6.927653279611684312, 6.477331591332402105, 39.20037568828259822 ) ) ;
#41695=EDGE_CURVE ( 'NONE', #7396, #8476, #24989, .T. ) ;
#41699=ORIENTED_EDGE ( 'NONE', *, *, #30097, .T. ) ;
#41708=CARTESIAN_POINT ( 'NONE',  ( 18.38992823210831773, 3.713927931064063159, 34.25328589890732900 ) ) ;
#41715=VERTEX_POINT ( 'NONE', #18388 ) ;
#41749=CARTESIAN_POINT ( 'NONE',  ( 4.257384923554909051, 0.7499999999999997780, 29.19375250200204164 ) ) ;
#41755=EDGE_CURVE ( 'NONE', #36959, #26221, #1696, .T. ) ;
#41756=DIRECTION ( 'NONE',  ( 0.000000000000000000, -1.000000000000000000, 0.000000000000000000 ) ) ;
#41775=CARTESIAN_POINT ( 'NONE',  ( -11.21606888246744127, -5.749999999999999112, 29.19375250200204519 ) ) ;
#41786=CARTESIAN_POINT ( 'NONE',  ( 33.00000000000001421, -10.75000000000000000, 32.19375250200202743 ) ) ;
#41823=AXIS2_PLACEMENT_3D ( 'NONE', #16449, #41982, #32800 ) ;
#41848=CIRCLE ( 'NONE', #9227, 6.999999999999992006 ) ;
#41975=DIRECTION ( 'NONE',  ( 0.000000000000000000, -1.000000000000000000, 0.000000000000000000 ) ) ;
#41982=DIRECTION ( 'NONE',  ( -0.000000000000000000, 1.000000000000000000, -0.000000000000000000 ) ) ;
#42011=LINE ( 'NONE', #16073, #32054 ) ;
#42013=CARTESIAN_POINT ( 'NONE',  ( 23.34627465269464253, 0.7499999999999997780, -52.99143003003683816 ) ) ;
#42031=ORIENTED_EDGE ( 'NONE', *, *, #36702, .F. ) ;
#42083=VERTEX_POINT ( 'NONE', #26870 ) ;
#42084=EDGE_CURVE ( 'NONE', #26548, #17635, #7817, .T. ) ;
#42094=VECTOR ( 'NONE', #30816, 1000.000000000000000 ) ;
#42095=CARTESIAN_POINT ( 'NONE',  ( 17.60377111545577478, 5.771009747771507215, 36.04897772278092560 ) ) ;
#42139=COLOUR_RGB('Sky Blue',0.24,0.69,0.87);
#42140=FILL_AREA_STYLE_COLOUR('',#42139);
#42141=FILL_AREA_STYLE('',(#42140));
#42142=SURFACE_STYLE_FILL_AREA(#42141);
#42143=SURFACE_SIDE_STYLE('',(#42142));
#42144=SURFACE_STYLE_USAGE(.BOTH.,#42143);
#42145=PRESENTATION_STYLE_ASSIGNMENT((#42144));
ENDSEC;
END-ISO-10303-21;
